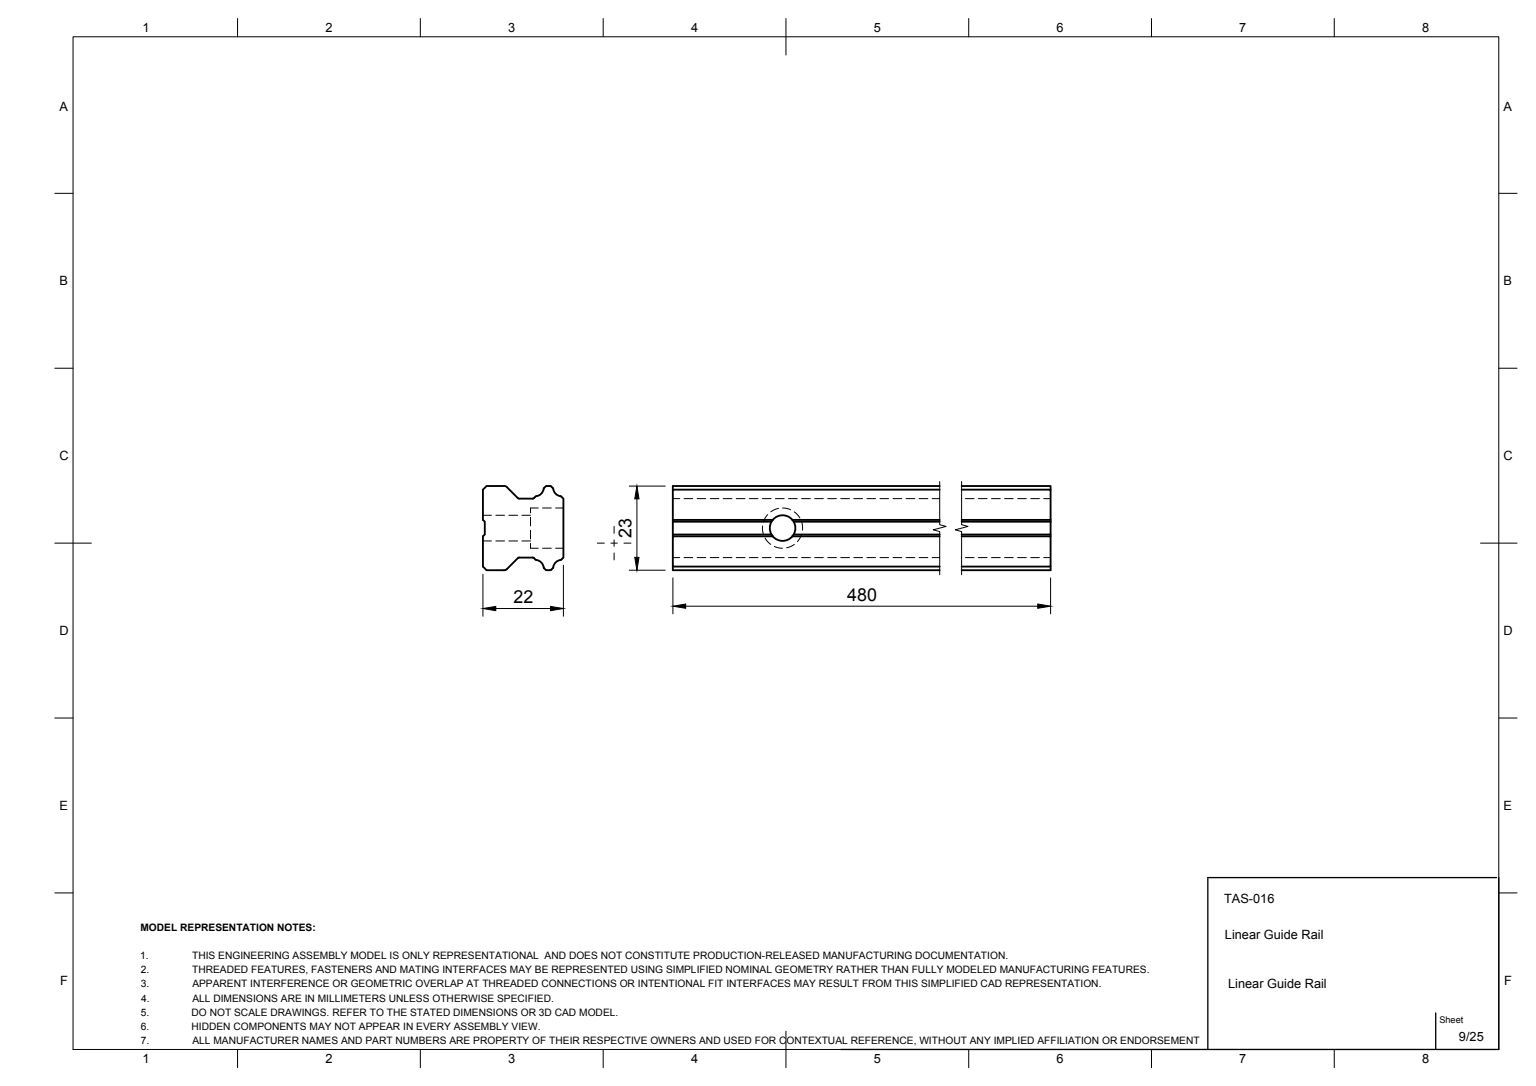
ISO-10303-21;
HEADER;
/* Generated by software containing ST-Developer
 * from STEP Tools, Inc. (www.steptools.com) 
 */

FILE_DESCRIPTION(
/* description */ ('STEP AP214'),
/* implementation_level */ '2;1');

FILE_NAME(
/* name */ 'Linear Guide Rail.step',
/* time_stamp */ '2026-11-15T14:55:55-08:00',
/* author */ (''),
/* organization */ (''),
/* preprocessor_version */ 'ST-DEVELOPER v20.2',
/* originating_system */ 'Autodesk Translation Framework v15.17.0.0',
/* authorisation */ '');

FILE_SCHEMA (('AUTOMOTIVE_DESIGN { 1 0 10303 214 3 1 1 }'));
ENDSEC;

DATA;
#10=MECHANICAL_DESIGN_GEOMETRIC_PRESENTATION_REPRESENTATION('',(#950),#57079);
#114=ELLIPSE('',#26276,4.9497474883957,3.50000001766466);
#115=ELLIPSE('',#26278,4.94974741758553,3.49999995496242);
#116=ELLIPSE('',#26282,4.94974750818554,3.50000003555096);
#117=ELLIPSE('',#26284,4.94974744933131,3.49999998268176);
#118=ELLIPSE('',#26290,4.94974743847195,3.49999997330407);
#119=ELLIPSE('',#26292,4.94974746764793,3.49999999946363);
#120=ELLIPSE('',#26296,4.94974747154346,3.5000000033075);
#121=ELLIPSE('',#26298,4.94974753359465,3.50000005774664);
#122=ELLIPSE('',#26304,4.94974746728535,3.49999999928767);
#123=ELLIPSE('',#26306,4.94974746000982,3.49999999272862);
#124=ELLIPSE('',#26310,4.94974744948699,3.49999998336686);
#125=ELLIPSE('',#26312,4.9497474011199,3.49999994011925);
#126=ELLIPSE('',#26318,4.94974750261449,3.50000003056212);
#127=ELLIPSE('',#26320,4.94974746233448,3.49999999488305);
#128=ELLIPSE('',#26324,4.94974747444535,3.50000000488897);
#129=ELLIPSE('',#26326,4.94974745285853,3.49999998629991);
#130=ELLIPSE('',#26332,4.94974749221039,3.50000002143459);
#131=ELLIPSE('',#26334,4.9497474654289,3.49999999744574);
#132=ELLIPSE('',#26338,4.94974747038,3.50000000169763);
#133=ELLIPSE('',#26340,4.94974743335947,3.49999996885897);
#134=ELLIPSE('',#26346,4.94974746422059,3.499999996325);
#135=ELLIPSE('',#26348,4.94974747922217,3.50000000966916);
#136=ELLIPSE('',#26352,4.94974747015525,3.50000000157014);
#137=ELLIPSE('',#26354,4.94974745455791,3.49999998774097);
#138=ELLIPSE('',#26360,4.94974745967519,3.49999999228821);
#139=ELLIPSE('',#26362,4.94974747586437,3.5000000067607);
#140=ELLIPSE('',#26366,4.94974746928504,3.50000000078832);
#141=ELLIPSE('',#26368,4.94974746799383,3.4999999996985);
#142=ELLIPSE('',#26374,4.94974746841778,3.50000000010074);
#143=ELLIPSE('',#26376,4.94974746853704,3.50000000020677);
#144=ELLIPSE('',#26380,4.94974746848257,3.50000000010871);
#145=ELLIPSE('',#26382,4.94974746829098,3.50000000002092);
#888=SHAPE_REPRESENTATION_RELATIONSHIP('SRR','None',#57278,#917);
#917=ADVANCED_BREP_SHAPE_REPRESENTATION('',(#987),#57070);
#950=STYLED_ITEM('',(#57444),#987);
#987=MANIFOLD_SOLID_BREP('Body1',#24550);
#1277=FACE_BOUND('',#4629,.T.);
#1278=FACE_BOUND('',#4630,.T.);
#1279=FACE_BOUND('',#4631,.T.);
#1280=FACE_BOUND('',#4632,.T.);
#1281=FACE_BOUND('',#4633,.T.);
#1282=FACE_BOUND('',#4634,.T.);
#1283=FACE_BOUND('',#4635,.T.);
#1284=FACE_BOUND('',#4636,.T.);
#1285=FACE_BOUND('',#4675,.T.);
#1286=FACE_BOUND('',#4677,.T.);
#1287=FACE_BOUND('',#4679,.T.);
#1288=FACE_BOUND('',#4681,.T.);
#1289=FACE_BOUND('',#4683,.T.);
#1290=FACE_BOUND('',#4685,.T.);
#1291=FACE_BOUND('',#4687,.T.);
#1292=FACE_BOUND('',#4689,.T.);
#1730=PLANE('',#26383);
#1731=PLANE('',#26384);
#1732=PLANE('',#26385);
#1733=PLANE('',#26386);
#1734=PLANE('',#26387);
#1735=PLANE('',#26388);
#1736=PLANE('',#26389);
#1737=PLANE('',#26390);
#1738=PLANE('',#26391);
#1739=PLANE('',#26392);
#1740=PLANE('',#26393);
#1741=PLANE('',#26394);
#1742=PLANE('',#26395);
#1743=PLANE('',#26396);
#1744=PLANE('',#26397);
#1745=PLANE('',#26398);
#1746=PLANE('',#26399);
#1747=PLANE('',#26400);
#1748=PLANE('',#26401);
#1749=PLANE('',#26402);
#1750=PLANE('',#26403);
#1751=PLANE('',#26404);
#1752=PLANE('',#26405);
#1753=PLANE('',#26406);
#1754=PLANE('',#26407);
#1755=PLANE('',#26408);
#1756=PLANE('',#26409);
#1757=PLANE('',#26432);
#1758=PLANE('',#26455);
#1759=PLANE('',#26456);
#1760=PLANE('',#26457);
#1761=PLANE('',#26458);
#1762=PLANE('',#26459);
#1763=PLANE('',#26460);
#1764=PLANE('',#26461);
#1765=PLANE('',#26462);
#1766=PLANE('',#26463);
#1767=PLANE('',#26464);
#1768=PLANE('',#26465);
#1769=PLANE('',#26466);
#1770=PLANE('',#26467);
#1771=PLANE('',#26468);
#1772=PLANE('',#26480);
#1773=PLANE('',#26481);
#1774=PLANE('',#26482);
#1775=PLANE('',#26483);
#1776=PLANE('',#26484);
#1777=PLANE('',#26496);
#1778=PLANE('',#26497);
#1779=PLANE('',#26498);
#1780=PLANE('',#26499);
#1781=PLANE('',#26500);
#1782=PLANE('',#26501);
#1783=PLANE('',#26502);
#1784=PLANE('',#26503);
#1785=PLANE('',#26504);
#1786=PLANE('',#26505);
#1787=PLANE('',#26506);
#2926=FACE_OUTER_BOUND('',#4578,.T.);
#2927=FACE_OUTER_BOUND('',#4579,.T.);
#2928=FACE_OUTER_BOUND('',#4580,.T.);
#2929=FACE_OUTER_BOUND('',#4581,.T.);
#2930=FACE_OUTER_BOUND('',#4582,.T.);
#2931=FACE_OUTER_BOUND('',#4583,.T.);
#2932=FACE_OUTER_BOUND('',#4584,.T.);
#2933=FACE_OUTER_BOUND('',#4585,.T.);
#2934=FACE_OUTER_BOUND('',#4586,.T.);
#2935=FACE_OUTER_BOUND('',#4587,.T.);
#2936=FACE_OUTER_BOUND('',#4588,.T.);
#2937=FACE_OUTER_BOUND('',#4589,.T.);
#2938=FACE_OUTER_BOUND('',#4590,.T.);
#2939=FACE_OUTER_BOUND('',#4591,.T.);
#2940=FACE_OUTER_BOUND('',#4592,.T.);
#2941=FACE_OUTER_BOUND('',#4593,.T.);
#2942=FACE_OUTER_BOUND('',#4594,.T.);
#2943=FACE_OUTER_BOUND('',#4595,.T.);
#2944=FACE_OUTER_BOUND('',#4596,.T.);
#2945=FACE_OUTER_BOUND('',#4597,.T.);
#2946=FACE_OUTER_BOUND('',#4598,.T.);
#2947=FACE_OUTER_BOUND('',#4599,.T.);
#2948=FACE_OUTER_BOUND('',#4600,.T.);
#2949=FACE_OUTER_BOUND('',#4601,.T.);
#2950=FACE_OUTER_BOUND('',#4602,.T.);
#2951=FACE_OUTER_BOUND('',#4603,.T.);
#2952=FACE_OUTER_BOUND('',#4604,.T.);
#2953=FACE_OUTER_BOUND('',#4605,.T.);
#2954=FACE_OUTER_BOUND('',#4606,.T.);
#2955=FACE_OUTER_BOUND('',#4607,.T.);
#2956=FACE_OUTER_BOUND('',#4608,.T.);
#2957=FACE_OUTER_BOUND('',#4609,.T.);
#2958=FACE_OUTER_BOUND('',#4610,.T.);
#2959=FACE_OUTER_BOUND('',#4611,.T.);
#2960=FACE_OUTER_BOUND('',#4612,.T.);
#2961=FACE_OUTER_BOUND('',#4613,.T.);
#2962=FACE_OUTER_BOUND('',#4614,.T.);
#2963=FACE_OUTER_BOUND('',#4615,.T.);
#2964=FACE_OUTER_BOUND('',#4616,.T.);
#2965=FACE_OUTER_BOUND('',#4617,.T.);
#2966=FACE_OUTER_BOUND('',#4618,.T.);
#2967=FACE_OUTER_BOUND('',#4619,.T.);
#2968=FACE_OUTER_BOUND('',#4620,.T.);
#2969=FACE_OUTER_BOUND('',#4621,.T.);
#2970=FACE_OUTER_BOUND('',#4622,.T.);
#2971=FACE_OUTER_BOUND('',#4623,.T.);
#2972=FACE_OUTER_BOUND('',#4624,.T.);
#2973=FACE_OUTER_BOUND('',#4625,.T.);
#2974=FACE_OUTER_BOUND('',#4626,.T.);
#2975=FACE_OUTER_BOUND('',#4627,.T.);
#2976=FACE_OUTER_BOUND('',#4628,.T.);
#2977=FACE_OUTER_BOUND('',#4637,.T.);
#2978=FACE_OUTER_BOUND('',#4638,.T.);
#2979=FACE_OUTER_BOUND('',#4639,.T.);
#2980=FACE_OUTER_BOUND('',#4640,.T.);
#2981=FACE_OUTER_BOUND('',#4641,.T.);
#2982=FACE_OUTER_BOUND('',#4642,.T.);
#2983=FACE_OUTER_BOUND('',#4643,.T.);
#2984=FACE_OUTER_BOUND('',#4644,.T.);
#2985=FACE_OUTER_BOUND('',#4645,.T.);
#2986=FACE_OUTER_BOUND('',#4646,.T.);
#2987=FACE_OUTER_BOUND('',#4647,.T.);
#2988=FACE_OUTER_BOUND('',#4648,.T.);
#2989=FACE_OUTER_BOUND('',#4649,.T.);
#2990=FACE_OUTER_BOUND('',#4650,.T.);
#2991=FACE_OUTER_BOUND('',#4651,.T.);
#2992=FACE_OUTER_BOUND('',#4652,.T.);
#2993=FACE_OUTER_BOUND('',#4653,.T.);
#2994=FACE_OUTER_BOUND('',#4654,.T.);
#2995=FACE_OUTER_BOUND('',#4655,.T.);
#2996=FACE_OUTER_BOUND('',#4656,.T.);
#2997=FACE_OUTER_BOUND('',#4657,.T.);
#2998=FACE_OUTER_BOUND('',#4658,.T.);
#2999=FACE_OUTER_BOUND('',#4659,.T.);
#3000=FACE_OUTER_BOUND('',#4660,.T.);
#3001=FACE_OUTER_BOUND('',#4661,.T.);
#3002=FACE_OUTER_BOUND('',#4662,.T.);
#3003=FACE_OUTER_BOUND('',#4663,.T.);
#3004=FACE_OUTER_BOUND('',#4664,.T.);
#3005=FACE_OUTER_BOUND('',#4665,.T.);
#3006=FACE_OUTER_BOUND('',#4666,.T.);
#3007=FACE_OUTER_BOUND('',#4667,.T.);
#3008=FACE_OUTER_BOUND('',#4668,.T.);
#3009=FACE_OUTER_BOUND('',#4669,.T.);
#3010=FACE_OUTER_BOUND('',#4670,.T.);
#3011=FACE_OUTER_BOUND('',#4671,.T.);
#3012=FACE_OUTER_BOUND('',#4672,.T.);
#3013=FACE_OUTER_BOUND('',#4673,.T.);
#3014=FACE_OUTER_BOUND('',#4674,.T.);
#3015=FACE_OUTER_BOUND('',#4676,.T.);
#3016=FACE_OUTER_BOUND('',#4678,.T.);
#3017=FACE_OUTER_BOUND('',#4680,.T.);
#3018=FACE_OUTER_BOUND('',#4682,.T.);
#3019=FACE_OUTER_BOUND('',#4684,.T.);
#3020=FACE_OUTER_BOUND('',#4686,.T.);
#3021=FACE_OUTER_BOUND('',#4688,.T.);
#4578=EDGE_LOOP('',(#19528,#19529,#19530,#19531));
#4579=EDGE_LOOP('',(#19532,#19533,#19534,#19535,#19536,#19537,#19538,#19539,
#19540,#19541,#19542,#19543));
#4580=EDGE_LOOP('',(#19544,#19545,#19546,#19547));
#4581=EDGE_LOOP('',(#19548,#19549,#19550,#19551,#19552,#19553,#19554,#19555,
#19556,#19557,#19558,#19559));
#4582=EDGE_LOOP('',(#19560,#19561,#19562,#19563));
#4583=EDGE_LOOP('',(#19564,#19565,#19566,#19567,#19568,#19569,#19570,#19571,
#19572,#19573,#19574,#19575));
#4584=EDGE_LOOP('',(#19576,#19577,#19578,#19579));
#4585=EDGE_LOOP('',(#19580,#19581,#19582,#19583,#19584,#19585,#19586,#19587,
#19588,#19589,#19590,#19591));
#4586=EDGE_LOOP('',(#19592,#19593,#19594,#19595));
#4587=EDGE_LOOP('',(#19596,#19597,#19598,#19599,#19600,#19601,#19602,#19603,
#19604,#19605,#19606,#19607));
#4588=EDGE_LOOP('',(#19608,#19609,#19610,#19611));
#4589=EDGE_LOOP('',(#19612,#19613,#19614,#19615,#19616,#19617,#19618,#19619,
#19620,#19621,#19622,#19623));
#4590=EDGE_LOOP('',(#19624,#19625,#19626,#19627));
#4591=EDGE_LOOP('',(#19628,#19629,#19630,#19631,#19632,#19633,#19634,#19635,
#19636,#19637,#19638,#19639));
#4592=EDGE_LOOP('',(#19640,#19641,#19642,#19643));
#4593=EDGE_LOOP('',(#19644,#19645,#19646,#19647,#19648,#19649,#19650,#19651,
#19652,#19653,#19654,#19655));
#4594=EDGE_LOOP('',(#19656,#19657,#19658,#19659));
#4595=EDGE_LOOP('',(#19660,#19661,#19662,#19663,#19664));
#4596=EDGE_LOOP('',(#19665,#19666,#19667,#19668));
#4597=EDGE_LOOP('',(#19669,#19670,#19671,#19672,#19673,#19674,#19675,#19676,
#19677,#19678,#19679,#19680,#19681,#19682,#19683,#19684,#19685,#19686,#19687,
#19688));
#4598=EDGE_LOOP('',(#19689,#19690,#19691,#19692,#19693,#19694,#19695,#19696,
#19697,#19698,#19699,#19700,#19701,#19702,#19703,#19704,#19705,#19706,#19707,
#19708));
#4599=EDGE_LOOP('',(#19709,#19710,#19711,#19712));
#4600=EDGE_LOOP('',(#19713,#19714,#19715,#19716,#19717));
#4601=EDGE_LOOP('',(#19718,#19719,#19720,#19721));
#4602=EDGE_LOOP('',(#19722,#19723,#19724,#19725));
#4603=EDGE_LOOP('',(#19726,#19727,#19728,#19729,#19730));
#4604=EDGE_LOOP('',(#19731,#19732,#19733,#19734));
#4605=EDGE_LOOP('',(#19735,#19736,#19737,#19738));
#4606=EDGE_LOOP('',(#19739,#19740,#19741,#19742));
#4607=EDGE_LOOP('',(#19743,#19744,#19745,#19746,#19747));
#4608=EDGE_LOOP('',(#19748,#19749,#19750,#19751));
#4609=EDGE_LOOP('',(#19752,#19753,#19754,#19755,#19756));
#4610=EDGE_LOOP('',(#19757,#19758,#19759,#19760));
#4611=EDGE_LOOP('',(#19761,#19762,#19763,#19764));
#4612=EDGE_LOOP('',(#19765,#19766,#19767,#19768,#19769));
#4613=EDGE_LOOP('',(#19770,#19771,#19772,#19773));
#4614=EDGE_LOOP('',(#19774,#19775,#19776,#19777));
#4615=EDGE_LOOP('',(#19778,#19779,#19780,#19781,#19782));
#4616=EDGE_LOOP('',(#19783,#19784,#19785,#19786));
#4617=EDGE_LOOP('',(#19787,#19788,#19789,#19790));
#4618=EDGE_LOOP('',(#19791,#19792,#19793,#19794));
#4619=EDGE_LOOP('',(#19795,#19796,#19797,#19798));
#4620=EDGE_LOOP('',(#19799,#19800,#19801,#19802,#19803,#19804,#19805,#19806,
#19807,#19808,#19809,#19810,#19811,#19812,#19813,#19814,#19815,#19816,#19817,
#19818,#19819,#19820,#19821,#19822,#19823,#19824,#19825,#19826,#19827,#19828,
#19829,#19830,#19831,#19832,#19833,#19834,#19835,#19836,#19837,#19838,#19839,
#19840,#19841,#19842,#19843,#19844));
#4621=EDGE_LOOP('',(#19845,#19846,#19847,#19848,#19849,#19850,#19851,#19852,
#19853,#19854,#19855,#19856,#19857,#19858,#19859,#19860,#19861,#19862,#19863,
#19864,#19865,#19866,#19867,#19868,#19869,#19870,#19871,#19872,#19873,#19874,
#19875,#19876,#19877,#19878,#19879,#19880,#19881,#19882,#19883,#19884,#19885,
#19886,#19887,#19888,#19889,#19890));
#4622=EDGE_LOOP('',(#19891,#19892,#19893,#19894));
#4623=EDGE_LOOP('',(#19895,#19896,#19897,#19898));
#4624=EDGE_LOOP('',(#19899,#19900,#19901,#19902));
#4625=EDGE_LOOP('',(#19903,#19904,#19905,#19906));
#4626=EDGE_LOOP('',(#19907,#19908,#19909,#19910));
#4627=EDGE_LOOP('',(#19911,#19912,#19913,#19914));
#4628=EDGE_LOOP('',(#19915,#19916,#19917,#19918));
#4629=EDGE_LOOP('',(#19919));
#4630=EDGE_LOOP('',(#19920));
#4631=EDGE_LOOP('',(#19921));
#4632=EDGE_LOOP('',(#19922));
#4633=EDGE_LOOP('',(#19923));
#4634=EDGE_LOOP('',(#19924));
#4635=EDGE_LOOP('',(#19925));
#4636=EDGE_LOOP('',(#19926));
#4637=EDGE_LOOP('',(#19927,#19928,#19929,#19930));
#4638=EDGE_LOOP('',(#19931,#19932,#19933,#19934));
#4639=EDGE_LOOP('',(#19935,#19936,#19937,#19938));
#4640=EDGE_LOOP('',(#19939,#19940,#19941,#19942));
#4641=EDGE_LOOP('',(#19943,#19944,#19945,#19946));
#4642=EDGE_LOOP('',(#19947,#19948,#19949,#19950));
#4643=EDGE_LOOP('',(#19951,#19952,#19953,#19954));
#4644=EDGE_LOOP('',(#19955,#19956,#19957,#19958));
#4645=EDGE_LOOP('',(#19959,#19960,#19961,#19962));
#4646=EDGE_LOOP('',(#19963,#19964,#19965,#19966));
#4647=EDGE_LOOP('',(#19967,#19968,#19969,#19970));
#4648=EDGE_LOOP('',(#19971,#19972,#19973,#19974));
#4649=EDGE_LOOP('',(#19975,#19976,#19977,#19978));
#4650=EDGE_LOOP('',(#19979,#19980,#19981,#19982));
#4651=EDGE_LOOP('',(#19983,#19984,#19985,#19986));
#4652=EDGE_LOOP('',(#19987,#19988,#19989,#19990));
#4653=EDGE_LOOP('',(#19991,#19992,#19993,#19994));
#4654=EDGE_LOOP('',(#19995,#19996,#19997,#19998));
#4655=EDGE_LOOP('',(#19999,#20000,#20001,#20002));
#4656=EDGE_LOOP('',(#20003,#20004,#20005,#20006));
#4657=EDGE_LOOP('',(#20007,#20008,#20009,#20010));
#4658=EDGE_LOOP('',(#20011,#20012,#20013,#20014));
#4659=EDGE_LOOP('',(#20015,#20016,#20017,#20018));
#4660=EDGE_LOOP('',(#20019,#20020,#20021,#20022));
#4661=EDGE_LOOP('',(#20023,#20024,#20025,#20026));
#4662=EDGE_LOOP('',(#20027,#20028,#20029,#20030));
#4663=EDGE_LOOP('',(#20031,#20032,#20033,#20034));
#4664=EDGE_LOOP('',(#20035,#20036,#20037,#20038));
#4665=EDGE_LOOP('',(#20039,#20040,#20041,#20042));
#4666=EDGE_LOOP('',(#20043,#20044,#20045,#20046));
#4667=EDGE_LOOP('',(#20047,#20048,#20049,#20050));
#4668=EDGE_LOOP('',(#20051,#20052,#20053,#20054));
#4669=EDGE_LOOP('',(#20055,#20056,#20057,#20058));
#4670=EDGE_LOOP('',(#20059,#20060,#20061,#20062));
#4671=EDGE_LOOP('',(#20063,#20064,#20065,#20066));
#4672=EDGE_LOOP('',(#20067,#20068,#20069,#20070,#20071));
#4673=EDGE_LOOP('',(#20072,#20073,#20074,#20075));
#4674=EDGE_LOOP('',(#20076));
#4675=EDGE_LOOP('',(#20077));
#4676=EDGE_LOOP('',(#20078));
#4677=EDGE_LOOP('',(#20079));
#4678=EDGE_LOOP('',(#20080));
#4679=EDGE_LOOP('',(#20081));
#4680=EDGE_LOOP('',(#20082));
#4681=EDGE_LOOP('',(#20083));
#4682=EDGE_LOOP('',(#20084));
#4683=EDGE_LOOP('',(#20085));
#4684=EDGE_LOOP('',(#20086));
#4685=EDGE_LOOP('',(#20087));
#4686=EDGE_LOOP('',(#20088));
#4687=EDGE_LOOP('',(#20089));
#4688=EDGE_LOOP('',(#20090));
#4689=EDGE_LOOP('',(#20091));
#6163=LINE('',#53474,#8130);
#6164=LINE('',#53489,#8131);
#6165=LINE('',#53502,#8132);
#6166=LINE('',#53517,#8133);
#6167=LINE('',#53530,#8134);
#6168=LINE('',#53545,#8135);
#6169=LINE('',#53558,#8136);
#6170=LINE('',#53573,#8137);
#6171=LINE('',#53586,#8138);
#6172=LINE('',#53601,#8139);
#6173=LINE('',#53614,#8140);
#6174=LINE('',#53629,#8141);
#6175=LINE('',#53642,#8142);
#6176=LINE('',#53657,#8143);
#6177=LINE('',#53670,#8144);
#6178=LINE('',#53685,#8145);
#6179=LINE('',#53696,#8146);
#6180=LINE('',#53698,#8147);
#6181=LINE('',#53699,#8148);
#6182=LINE('',#53701,#8149);
#6183=LINE('',#53702,#8150);
#6184=LINE('',#53704,#8151);
#6185=LINE('',#53706,#8152);
#6186=LINE('',#53707,#8153);
#6187=LINE('',#53708,#8154);
#6188=LINE('',#53709,#8155);
#6189=LINE('',#53710,#8156);
#6190=LINE('',#53711,#8157);
#6191=LINE('',#53712,#8158);
#6192=LINE('',#53714,#8159);
#6193=LINE('',#53716,#8160);
#6194=LINE('',#53718,#8161);
#6195=LINE('',#53719,#8162);
#6196=LINE('',#53722,#8163);
#6197=LINE('',#53724,#8164);
#6198=LINE('',#53726,#8165);
#6199=LINE('',#53728,#8166);
#6200=LINE('',#53729,#8167);
#6201=LINE('',#53730,#8168);
#6202=LINE('',#53731,#8169);
#6203=LINE('',#53732,#8170);
#6204=LINE('',#53733,#8171);
#6205=LINE('',#53734,#8172);
#6206=LINE('',#53735,#8173);
#6207=LINE('',#53738,#8174);
#6208=LINE('',#53739,#8175);
#6209=LINE('',#53743,#8176);
#6210=LINE('',#53744,#8177);
#6211=LINE('',#53748,#8178);
#6212=LINE('',#53750,#8179);
#6213=LINE('',#53753,#8180);
#6214=LINE('',#53754,#8181);
#6215=LINE('',#53758,#8182);
#6216=LINE('',#53759,#8183);
#6217=LINE('',#53763,#8184);
#6218=LINE('',#53764,#8185);
#6219=LINE('',#53769,#8186);
#6220=LINE('',#53771,#8187);
#6221=LINE('',#53772,#8188);
#6222=LINE('',#53774,#8189);
#6223=LINE('',#53777,#8190);
#6224=LINE('',#53779,#8191);
#6225=LINE('',#53783,#8192);
#6226=LINE('',#53787,#8193);
#6227=LINE('',#53791,#8194);
#6228=LINE('',#53799,#8195);
#6229=LINE('',#53803,#8196);
#6230=LINE('',#53807,#8197);
#6231=LINE('',#53815,#8198);
#6232=LINE('',#53817,#8199);
#6233=LINE('',#53819,#8200);
#6234=LINE('',#53827,#8201);
#6235=LINE('',#53831,#8202);
#6236=LINE('',#53835,#8203);
#6237=LINE('',#53843,#8204);
#6238=LINE('',#53847,#8205);
#6239=LINE('',#53851,#8206);
#6240=LINE('',#53855,#8207);
#6241=LINE('',#53856,#8208);
#6242=LINE('',#53858,#8209);
#6243=LINE('',#53859,#8210);
#6244=LINE('',#53861,#8211);
#6245=LINE('',#53863,#8212);
#6246=LINE('',#53865,#8213);
#6247=LINE('',#53869,#8214);
#6248=LINE('',#53873,#8215);
#6249=LINE('',#53877,#8216);
#6250=LINE('',#53885,#8217);
#6251=LINE('',#53889,#8218);
#6252=LINE('',#53893,#8219);
#6253=LINE('',#53901,#8220);
#6254=LINE('',#53903,#8221);
#6255=LINE('',#53905,#8222);
#6256=LINE('',#53913,#8223);
#6257=LINE('',#53917,#8224);
#6258=LINE('',#53921,#8225);
#6259=LINE('',#53929,#8226);
#6260=LINE('',#53933,#8227);
#6261=LINE('',#53937,#8228);
#6262=LINE('',#53941,#8229);
#6263=LINE('',#53942,#8230);
#6264=LINE('',#53944,#8231);
#6265=LINE('',#53945,#8232);
#6266=LINE('',#53947,#8233);
#6267=LINE('',#53948,#8234);
#6268=LINE('',#53950,#8235);
#6269=LINE('',#53951,#8236);
#6270=LINE('',#53953,#8237);
#6271=LINE('',#53954,#8238);
#6272=LINE('',#53956,#8239);
#6273=LINE('',#53957,#8240);
#6274=LINE('',#53959,#8241);
#6275=LINE('',#53960,#8242);
#6276=LINE('',#53962,#8243);
#6277=LINE('',#53964,#8244);
#6278=LINE('',#53966,#8245);
#6279=LINE('',#53968,#8246);
#6280=LINE('',#53969,#8247);
#6281=LINE('',#53971,#8248);
#6282=LINE('',#53972,#8249);
#6283=LINE('',#53974,#8250);
#6284=LINE('',#53975,#8251);
#6285=LINE('',#53977,#8252);
#6286=LINE('',#53978,#8253);
#6287=LINE('',#53980,#8254);
#6288=LINE('',#53982,#8255);
#6289=LINE('',#53983,#8256);
#6290=LINE('',#53985,#8257);
#6291=LINE('',#53986,#8258);
#6292=LINE('',#53997,#8259);
#6293=LINE('',#53998,#8260);
#6294=LINE('',#54000,#8261);
#6295=LINE('',#54001,#8262);
#6296=LINE('',#54003,#8263);
#6297=LINE('',#54004,#8264);
#6298=LINE('',#54006,#8265);
#6299=LINE('',#54007,#8266);
#6300=LINE('',#54010,#8267);
#6301=LINE('',#54011,#8268);
#6302=LINE('',#54013,#8269);
#6303=LINE('',#54014,#8270);
#6304=LINE('',#54026,#8271);
#8130=VECTOR('',#31169,5.50000000000001);
#8131=VECTOR('',#31184,3.5);
#8132=VECTOR('',#31199,5.50000000000001);
#8133=VECTOR('',#31214,3.5);
#8134=VECTOR('',#31229,5.50000000000001);
#8135=VECTOR('',#31244,3.5);
#8136=VECTOR('',#31259,5.50000000000001);
#8137=VECTOR('',#31274,3.5);
#8138=VECTOR('',#31289,5.50000000000001);
#8139=VECTOR('',#31304,3.5);
#8140=VECTOR('',#31319,5.50000000000001);
#8141=VECTOR('',#31334,3.5);
#8142=VECTOR('',#31349,5.5);
#8143=VECTOR('',#31364,3.5);
#8144=VECTOR('',#31379,5.5);
#8145=VECTOR('',#31394,3.5);
#8146=VECTOR('',#31407,1000.);
#8147=VECTOR('',#31408,1000.);
#8148=VECTOR('',#31409,1000.);
#8149=VECTOR('',#31412,1000.);
#8150=VECTOR('',#31413,1000.);
#8151=VECTOR('',#31416,1000.);
#8152=VECTOR('',#31419,1000.);
#8153=VECTOR('',#31420,1000.);
#8154=VECTOR('',#31421,1000.);
#8155=VECTOR('',#31422,1000.);
#8156=VECTOR('',#31423,1000.);
#8157=VECTOR('',#31424,1000.);
#8158=VECTOR('',#31425,1000.);
#8159=VECTOR('',#31426,1000.);
#8160=VECTOR('',#31427,1000.);
#8161=VECTOR('',#31428,1000.);
#8162=VECTOR('',#31429,1000.);
#8163=VECTOR('',#31432,1000.);
#8164=VECTOR('',#31433,1000.);
#8165=VECTOR('',#31434,1000.);
#8166=VECTOR('',#31435,1000.);
#8167=VECTOR('',#31436,1000.);
#8168=VECTOR('',#31437,1000.);
#8169=VECTOR('',#31438,1000.);
#8170=VECTOR('',#31439,1000.);
#8171=VECTOR('',#31440,1000.);
#8172=VECTOR('',#31441,1000.);
#8173=VECTOR('',#31442,1000.);
#8174=VECTOR('',#31447,1000.);
#8175=VECTOR('',#31448,1000.);
#8176=VECTOR('',#31455,1000.);
#8177=VECTOR('',#31456,1000.);
#8178=VECTOR('',#31463,1000.);
#8179=VECTOR('',#31466,1000.);
#8180=VECTOR('',#31471,1000.);
#8181=VECTOR('',#31472,1000.);
#8182=VECTOR('',#31479,1000.);
#8183=VECTOR('',#31480,1000.);
#8184=VECTOR('',#31487,1000.);
#8185=VECTOR('',#31488,1000.);
#8186=VECTOR('',#31495,1000.);
#8187=VECTOR('',#31496,1000.);
#8188=VECTOR('',#31497,1000.);
#8189=VECTOR('',#31500,1000.);
#8190=VECTOR('',#31503,1000.);
#8191=VECTOR('',#31504,1000.);
#8192=VECTOR('',#31507,1000.);
#8193=VECTOR('',#31510,1000.);
#8194=VECTOR('',#31513,1000.);
#8195=VECTOR('',#31520,1000.);
#8196=VECTOR('',#31523,1000.);
#8197=VECTOR('',#31526,1000.);
#8198=VECTOR('',#31533,1000.);
#8199=VECTOR('',#31534,1000.);
#8200=VECTOR('',#31535,1000.);
#8201=VECTOR('',#31542,1000.);
#8202=VECTOR('',#31545,1000.);
#8203=VECTOR('',#31548,1000.);
#8204=VECTOR('',#31555,1000.);
#8205=VECTOR('',#31558,1000.);
#8206=VECTOR('',#31561,1000.);
#8207=VECTOR('',#31564,1000.);
#8208=VECTOR('',#31565,1000.);
#8209=VECTOR('',#31566,1000.);
#8210=VECTOR('',#31567,1000.);
#8211=VECTOR('',#31570,1000.);
#8212=VECTOR('',#31571,1000.);
#8213=VECTOR('',#31572,1000.);
#8214=VECTOR('',#31575,1000.);
#8215=VECTOR('',#31578,1000.);
#8216=VECTOR('',#31581,1000.);
#8217=VECTOR('',#31588,1000.);
#8218=VECTOR('',#31591,1000.);
#8219=VECTOR('',#31594,1000.);
#8220=VECTOR('',#31601,1000.);
#8221=VECTOR('',#31602,1000.);
#8222=VECTOR('',#31603,1000.);
#8223=VECTOR('',#31610,1000.);
#8224=VECTOR('',#31613,1000.);
#8225=VECTOR('',#31616,1000.);
#8226=VECTOR('',#31623,1000.);
#8227=VECTOR('',#31626,1000.);
#8228=VECTOR('',#31629,1000.);
#8229=VECTOR('',#31632,1000.);
#8230=VECTOR('',#31633,1000.);
#8231=VECTOR('',#31636,1000.);
#8232=VECTOR('',#31637,1000.);
#8233=VECTOR('',#31640,1000.);
#8234=VECTOR('',#31641,1000.);
#8235=VECTOR('',#31644,1000.);
#8236=VECTOR('',#31645,1000.);
#8237=VECTOR('',#31648,1000.);
#8238=VECTOR('',#31649,1000.);
#8239=VECTOR('',#31652,1000.);
#8240=VECTOR('',#31653,1000.);
#8241=VECTOR('',#31656,1000.);
#8242=VECTOR('',#31657,1000.);
#8243=VECTOR('',#31660,1000.);
#8244=VECTOR('',#31663,1000.);
#8245=VECTOR('',#31666,1000.);
#8246=VECTOR('',#31669,1000.);
#8247=VECTOR('',#31670,1000.);
#8248=VECTOR('',#31673,1000.);
#8249=VECTOR('',#31674,1000.);
#8250=VECTOR('',#31677,1000.);
#8251=VECTOR('',#31678,1000.);
#8252=VECTOR('',#31681,1000.);
#8253=VECTOR('',#31682,1000.);
#8254=VECTOR('',#31685,1000.);
#8255=VECTOR('',#31688,1000.);
#8256=VECTOR('',#31689,1000.);
#8257=VECTOR('',#31692,1000.);
#8258=VECTOR('',#31693,1000.);
#8259=VECTOR('',#31714,1000.);
#8260=VECTOR('',#31715,1000.);
#8261=VECTOR('',#31718,1000.);
#8262=VECTOR('',#31719,1000.);
#8263=VECTOR('',#31722,1000.);
#8264=VECTOR('',#31723,1000.);
#8265=VECTOR('',#31726,1000.);
#8266=VECTOR('',#31727,1000.);
#8267=VECTOR('',#31732,1000.);
#8268=VECTOR('',#31733,1000.);
#8269=VECTOR('',#31736,1000.);
#8270=VECTOR('',#31737,1000.);
#8271=VECTOR('',#31760,1000.);
#9808=CIRCLE('',#26272,5.50000000000001);
#9809=CIRCLE('',#26273,5.50000000000001);
#9810=CIRCLE('',#26275,3.5);
#9811=CIRCLE('',#26277,3.5);
#9812=CIRCLE('',#26279,3.5);
#9813=CIRCLE('',#26280,3.5);
#9814=CIRCLE('',#26281,3.5);
#9815=CIRCLE('',#26283,3.5);
#9816=CIRCLE('',#26286,5.50000000000001);
#9817=CIRCLE('',#26287,5.50000000000001);
#9818=CIRCLE('',#26289,3.5);
#9819=CIRCLE('',#26291,3.5);
#9820=CIRCLE('',#26293,3.5);
#9821=CIRCLE('',#26294,3.5);
#9822=CIRCLE('',#26295,3.5);
#9823=CIRCLE('',#26297,3.5);
#9824=CIRCLE('',#26300,5.50000000000001);
#9825=CIRCLE('',#26301,5.50000000000001);
#9826=CIRCLE('',#26303,3.5);
#9827=CIRCLE('',#26305,3.5);
#9828=CIRCLE('',#26307,3.5);
#9829=CIRCLE('',#26308,3.5);
#9830=CIRCLE('',#26309,3.5);
#9831=CIRCLE('',#26311,3.5);
#9832=CIRCLE('',#26314,5.50000000000001);
#9833=CIRCLE('',#26315,5.50000000000001);
#9834=CIRCLE('',#26317,3.5);
#9835=CIRCLE('',#26319,3.5);
#9836=CIRCLE('',#26321,3.5);
#9837=CIRCLE('',#26322,3.5);
#9838=CIRCLE('',#26323,3.5);
#9839=CIRCLE('',#26325,3.5);
#9840=CIRCLE('',#26328,5.50000000000001);
#9841=CIRCLE('',#26329,5.50000000000001);
#9842=CIRCLE('',#26331,3.5);
#9843=CIRCLE('',#26333,3.5);
#9844=CIRCLE('',#26335,3.5);
#9845=CIRCLE('',#26336,3.5);
#9846=CIRCLE('',#26337,3.5);
#9847=CIRCLE('',#26339,3.5);
#9848=CIRCLE('',#26342,5.50000000000001);
#9849=CIRCLE('',#26343,5.50000000000001);
#9850=CIRCLE('',#26345,3.5);
#9851=CIRCLE('',#26347,3.49999999999999);
#9852=CIRCLE('',#26349,3.5);
#9853=CIRCLE('',#26350,3.5);
#9854=CIRCLE('',#26351,3.5);
#9855=CIRCLE('',#26353,3.49999999999999);
#9856=CIRCLE('',#26356,5.5);
#9857=CIRCLE('',#26357,5.5);
#9858=CIRCLE('',#26359,3.5);
#9859=CIRCLE('',#26361,3.5);
#9860=CIRCLE('',#26363,3.5);
#9861=CIRCLE('',#26364,3.5);
#9862=CIRCLE('',#26365,3.5);
#9863=CIRCLE('',#26367,3.5);
#9864=CIRCLE('',#26370,5.5);
#9865=CIRCLE('',#26371,5.5);
#9866=CIRCLE('',#26373,3.5);
#9867=CIRCLE('',#26375,3.49999999999999);
#9868=CIRCLE('',#26377,3.5);
#9869=CIRCLE('',#26378,3.5);
#9870=CIRCLE('',#26379,3.5);
#9871=CIRCLE('',#26381,3.49999999999999);
#9872=CIRCLE('',#26410,0.999999999999999);
#9873=CIRCLE('',#26411,0.5);
#9874=CIRCLE('',#26412,0.5);
#9875=CIRCLE('',#26413,0.5);
#9876=CIRCLE('',#26414,2.3);
#9877=CIRCLE('',#26415,0.5);
#9878=CIRCLE('',#26416,0.5);
#9879=CIRCLE('',#26417,0.5);
#9880=CIRCLE('',#26418,0.5);
#9881=CIRCLE('',#26419,2.3);
#9882=CIRCLE('',#26420,0.5);
#9883=CIRCLE('',#26421,0.5);
#9884=CIRCLE('',#26422,2.3);
#9885=CIRCLE('',#26423,0.5);
#9886=CIRCLE('',#26424,0.5);
#9887=CIRCLE('',#26425,0.5);
#9888=CIRCLE('',#26426,0.5);
#9889=CIRCLE('',#26427,2.3);
#9890=CIRCLE('',#26428,0.5);
#9891=CIRCLE('',#26429,0.5);
#9892=CIRCLE('',#26430,0.5);
#9893=CIRCLE('',#26431,0.999999999999999);
#9894=CIRCLE('',#26433,0.999999999999999);
#9895=CIRCLE('',#26434,0.5);
#9896=CIRCLE('',#26435,0.5);
#9897=CIRCLE('',#26436,0.5);
#9898=CIRCLE('',#26437,2.3);
#9899=CIRCLE('',#26438,0.5);
#9900=CIRCLE('',#26439,0.5);
#9901=CIRCLE('',#26440,0.5);
#9902=CIRCLE('',#26441,0.5);
#9903=CIRCLE('',#26442,2.3);
#9904=CIRCLE('',#26443,0.5);
#9905=CIRCLE('',#26444,0.5);
#9906=CIRCLE('',#26445,2.3);
#9907=CIRCLE('',#26446,0.5);
#9908=CIRCLE('',#26447,0.5);
#9909=CIRCLE('',#26448,0.5);
#9910=CIRCLE('',#26449,0.5);
#9911=CIRCLE('',#26450,2.3);
#9912=CIRCLE('',#26451,0.5);
#9913=CIRCLE('',#26452,0.5);
#9914=CIRCLE('',#26453,0.5);
#9915=CIRCLE('',#26454,0.999999999999999);
#11441=VERTEX_POINT('',#53471);
#11442=VERTEX_POINT('',#53473);
#11443=VERTEX_POINT('',#53477);
#11444=VERTEX_POINT('',#53478);
#11445=VERTEX_POINT('',#53480);
#11446=VERTEX_POINT('',#53482);
#11447=VERTEX_POINT('',#53484);
#11448=VERTEX_POINT('',#53486);
#11449=VERTEX_POINT('',#53488);
#11450=VERTEX_POINT('',#53491);
#11451=VERTEX_POINT('',#53493);
#11452=VERTEX_POINT('',#53495);
#11453=VERTEX_POINT('',#53499);
#11454=VERTEX_POINT('',#53501);
#11455=VERTEX_POINT('',#53505);
#11456=VERTEX_POINT('',#53506);
#11457=VERTEX_POINT('',#53508);
#11458=VERTEX_POINT('',#53510);
#11459=VERTEX_POINT('',#53512);
#11460=VERTEX_POINT('',#53514);
#11461=VERTEX_POINT('',#53516);
#11462=VERTEX_POINT('',#53519);
#11463=VERTEX_POINT('',#53521);
#11464=VERTEX_POINT('',#53523);
#11465=VERTEX_POINT('',#53527);
#11466=VERTEX_POINT('',#53529);
#11467=VERTEX_POINT('',#53533);
#11468=VERTEX_POINT('',#53534);
#11469=VERTEX_POINT('',#53536);
#11470=VERTEX_POINT('',#53538);
#11471=VERTEX_POINT('',#53540);
#11472=VERTEX_POINT('',#53542);
#11473=VERTEX_POINT('',#53544);
#11474=VERTEX_POINT('',#53547);
#11475=VERTEX_POINT('',#53549);
#11476=VERTEX_POINT('',#53551);
#11477=VERTEX_POINT('',#53555);
#11478=VERTEX_POINT('',#53557);
#11479=VERTEX_POINT('',#53561);
#11480=VERTEX_POINT('',#53562);
#11481=VERTEX_POINT('',#53564);
#11482=VERTEX_POINT('',#53566);
#11483=VERTEX_POINT('',#53568);
#11484=VERTEX_POINT('',#53570);
#11485=VERTEX_POINT('',#53572);
#11486=VERTEX_POINT('',#53575);
#11487=VERTEX_POINT('',#53577);
#11488=VERTEX_POINT('',#53579);
#11489=VERTEX_POINT('',#53583);
#11490=VERTEX_POINT('',#53585);
#11491=VERTEX_POINT('',#53589);
#11492=VERTEX_POINT('',#53590);
#11493=VERTEX_POINT('',#53592);
#11494=VERTEX_POINT('',#53594);
#11495=VERTEX_POINT('',#53596);
#11496=VERTEX_POINT('',#53598);
#11497=VERTEX_POINT('',#53600);
#11498=VERTEX_POINT('',#53603);
#11499=VERTEX_POINT('',#53605);
#11500=VERTEX_POINT('',#53607);
#11501=VERTEX_POINT('',#53611);
#11502=VERTEX_POINT('',#53613);
#11503=VERTEX_POINT('',#53617);
#11504=VERTEX_POINT('',#53618);
#11505=VERTEX_POINT('',#53620);
#11506=VERTEX_POINT('',#53622);
#11507=VERTEX_POINT('',#53624);
#11508=VERTEX_POINT('',#53626);
#11509=VERTEX_POINT('',#53628);
#11510=VERTEX_POINT('',#53631);
#11511=VERTEX_POINT('',#53633);
#11512=VERTEX_POINT('',#53635);
#11513=VERTEX_POINT('',#53639);
#11514=VERTEX_POINT('',#53641);
#11515=VERTEX_POINT('',#53645);
#11516=VERTEX_POINT('',#53646);
#11517=VERTEX_POINT('',#53648);
#11518=VERTEX_POINT('',#53650);
#11519=VERTEX_POINT('',#53652);
#11520=VERTEX_POINT('',#53654);
#11521=VERTEX_POINT('',#53656);
#11522=VERTEX_POINT('',#53659);
#11523=VERTEX_POINT('',#53661);
#11524=VERTEX_POINT('',#53663);
#11525=VERTEX_POINT('',#53667);
#11526=VERTEX_POINT('',#53669);
#11527=VERTEX_POINT('',#53673);
#11528=VERTEX_POINT('',#53674);
#11529=VERTEX_POINT('',#53676);
#11530=VERTEX_POINT('',#53678);
#11531=VERTEX_POINT('',#53680);
#11532=VERTEX_POINT('',#53682);
#11533=VERTEX_POINT('',#53684);
#11534=VERTEX_POINT('',#53687);
#11535=VERTEX_POINT('',#53689);
#11536=VERTEX_POINT('',#53691);
#11537=VERTEX_POINT('',#53695);
#11538=VERTEX_POINT('',#53697);
#11539=VERTEX_POINT('',#53713);
#11540=VERTEX_POINT('',#53715);
#11541=VERTEX_POINT('',#53717);
#11542=VERTEX_POINT('',#53721);
#11543=VERTEX_POINT('',#53723);
#11544=VERTEX_POINT('',#53725);
#11545=VERTEX_POINT('',#53727);
#11546=VERTEX_POINT('',#53768);
#11547=VERTEX_POINT('',#53770);
#11548=VERTEX_POINT('',#53776);
#11549=VERTEX_POINT('',#53778);
#11550=VERTEX_POINT('',#53780);
#11551=VERTEX_POINT('',#53782);
#11552=VERTEX_POINT('',#53784);
#11553=VERTEX_POINT('',#53786);
#11554=VERTEX_POINT('',#53788);
#11555=VERTEX_POINT('',#53790);
#11556=VERTEX_POINT('',#53792);
#11557=VERTEX_POINT('',#53794);
#11558=VERTEX_POINT('',#53796);
#11559=VERTEX_POINT('',#53798);
#11560=VERTEX_POINT('',#53800);
#11561=VERTEX_POINT('',#53802);
#11562=VERTEX_POINT('',#53804);
#11563=VERTEX_POINT('',#53806);
#11564=VERTEX_POINT('',#53808);
#11565=VERTEX_POINT('',#53810);
#11566=VERTEX_POINT('',#53812);
#11567=VERTEX_POINT('',#53814);
#11568=VERTEX_POINT('',#53816);
#11569=VERTEX_POINT('',#53818);
#11570=VERTEX_POINT('',#53820);
#11571=VERTEX_POINT('',#53822);
#11572=VERTEX_POINT('',#53824);
#11573=VERTEX_POINT('',#53826);
#11574=VERTEX_POINT('',#53828);
#11575=VERTEX_POINT('',#53830);
#11576=VERTEX_POINT('',#53832);
#11577=VERTEX_POINT('',#53834);
#11578=VERTEX_POINT('',#53836);
#11579=VERTEX_POINT('',#53838);
#11580=VERTEX_POINT('',#53840);
#11581=VERTEX_POINT('',#53842);
#11582=VERTEX_POINT('',#53844);
#11583=VERTEX_POINT('',#53846);
#11584=VERTEX_POINT('',#53848);
#11585=VERTEX_POINT('',#53850);
#11586=VERTEX_POINT('',#53852);
#11587=VERTEX_POINT('',#53854);
#11588=VERTEX_POINT('',#53857);
#11589=VERTEX_POINT('',#53862);
#11590=VERTEX_POINT('',#53864);
#11591=VERTEX_POINT('',#53866);
#11592=VERTEX_POINT('',#53868);
#11593=VERTEX_POINT('',#53870);
#11594=VERTEX_POINT('',#53872);
#11595=VERTEX_POINT('',#53874);
#11596=VERTEX_POINT('',#53876);
#11597=VERTEX_POINT('',#53878);
#11598=VERTEX_POINT('',#53880);
#11599=VERTEX_POINT('',#53882);
#11600=VERTEX_POINT('',#53884);
#11601=VERTEX_POINT('',#53886);
#11602=VERTEX_POINT('',#53888);
#11603=VERTEX_POINT('',#53890);
#11604=VERTEX_POINT('',#53892);
#11605=VERTEX_POINT('',#53894);
#11606=VERTEX_POINT('',#53896);
#11607=VERTEX_POINT('',#53898);
#11608=VERTEX_POINT('',#53900);
#11609=VERTEX_POINT('',#53902);
#11610=VERTEX_POINT('',#53904);
#11611=VERTEX_POINT('',#53906);
#11612=VERTEX_POINT('',#53908);
#11613=VERTEX_POINT('',#53910);
#11614=VERTEX_POINT('',#53912);
#11615=VERTEX_POINT('',#53914);
#11616=VERTEX_POINT('',#53916);
#11617=VERTEX_POINT('',#53918);
#11618=VERTEX_POINT('',#53920);
#11619=VERTEX_POINT('',#53922);
#11620=VERTEX_POINT('',#53924);
#11621=VERTEX_POINT('',#53926);
#11622=VERTEX_POINT('',#53928);
#11623=VERTEX_POINT('',#53930);
#11624=VERTEX_POINT('',#53932);
#11625=VERTEX_POINT('',#53934);
#11626=VERTEX_POINT('',#53936);
#11627=VERTEX_POINT('',#53938);
#11628=VERTEX_POINT('',#53940);
#14309=EDGE_CURVE('',#11441,#11441,#9808,.T.);
#14310=EDGE_CURVE('',#11441,#11442,#6163,.T.);
#14311=EDGE_CURVE('',#11442,#11442,#9809,.T.);
#14312=EDGE_CURVE('',#11443,#11444,#9810,.T.);
#14313=EDGE_CURVE('',#11445,#11443,#114,.T.);
#14314=EDGE_CURVE('',#11446,#11445,#9811,.T.);
#14315=EDGE_CURVE('',#11447,#11446,#115,.T.);
#14316=EDGE_CURVE('',#11448,#11447,#9812,.T.);
#14317=EDGE_CURVE('',#11448,#11449,#6164,.T.);
#14318=EDGE_CURVE('',#11449,#11449,#9813,.T.);
#14319=EDGE_CURVE('',#11450,#11448,#9814,.T.);
#14320=EDGE_CURVE('',#11451,#11450,#116,.T.);
#14321=EDGE_CURVE('',#11452,#11451,#9815,.T.);
#14322=EDGE_CURVE('',#11444,#11452,#117,.T.);
#14323=EDGE_CURVE('',#11453,#11453,#9816,.T.);
#14324=EDGE_CURVE('',#11453,#11454,#6165,.T.);
#14325=EDGE_CURVE('',#11454,#11454,#9817,.T.);
#14326=EDGE_CURVE('',#11455,#11456,#9818,.T.);
#14327=EDGE_CURVE('',#11457,#11455,#118,.T.);
#14328=EDGE_CURVE('',#11458,#11457,#9819,.T.);
#14329=EDGE_CURVE('',#11459,#11458,#119,.T.);
#14330=EDGE_CURVE('',#11460,#11459,#9820,.T.);
#14331=EDGE_CURVE('',#11460,#11461,#6166,.T.);
#14332=EDGE_CURVE('',#11461,#11461,#9821,.T.);
#14333=EDGE_CURVE('',#11462,#11460,#9822,.T.);
#14334=EDGE_CURVE('',#11463,#11462,#120,.T.);
#14335=EDGE_CURVE('',#11464,#11463,#9823,.T.);
#14336=EDGE_CURVE('',#11456,#11464,#121,.T.);
#14337=EDGE_CURVE('',#11465,#11465,#9824,.T.);
#14338=EDGE_CURVE('',#11465,#11466,#6167,.T.);
#14339=EDGE_CURVE('',#11466,#11466,#9825,.T.);
#14340=EDGE_CURVE('',#11467,#11468,#9826,.T.);
#14341=EDGE_CURVE('',#11469,#11467,#122,.T.);
#14342=EDGE_CURVE('',#11470,#11469,#9827,.T.);
#14343=EDGE_CURVE('',#11471,#11470,#123,.T.);
#14344=EDGE_CURVE('',#11472,#11471,#9828,.T.);
#14345=EDGE_CURVE('',#11472,#11473,#6168,.T.);
#14346=EDGE_CURVE('',#11473,#11473,#9829,.T.);
#14347=EDGE_CURVE('',#11474,#11472,#9830,.T.);
#14348=EDGE_CURVE('',#11475,#11474,#124,.T.);
#14349=EDGE_CURVE('',#11476,#11475,#9831,.T.);
#14350=EDGE_CURVE('',#11468,#11476,#125,.T.);
#14351=EDGE_CURVE('',#11477,#11477,#9832,.T.);
#14352=EDGE_CURVE('',#11477,#11478,#6169,.T.);
#14353=EDGE_CURVE('',#11478,#11478,#9833,.T.);
#14354=EDGE_CURVE('',#11479,#11480,#9834,.T.);
#14355=EDGE_CURVE('',#11481,#11479,#126,.T.);
#14356=EDGE_CURVE('',#11482,#11481,#9835,.T.);
#14357=EDGE_CURVE('',#11483,#11482,#127,.T.);
#14358=EDGE_CURVE('',#11484,#11483,#9836,.T.);
#14359=EDGE_CURVE('',#11484,#11485,#6170,.T.);
#14360=EDGE_CURVE('',#11485,#11485,#9837,.T.);
#14361=EDGE_CURVE('',#11486,#11484,#9838,.T.);
#14362=EDGE_CURVE('',#11487,#11486,#128,.T.);
#14363=EDGE_CURVE('',#11488,#11487,#9839,.T.);
#14364=EDGE_CURVE('',#11480,#11488,#129,.T.);
#14365=EDGE_CURVE('',#11489,#11489,#9840,.T.);
#14366=EDGE_CURVE('',#11489,#11490,#6171,.T.);
#14367=EDGE_CURVE('',#11490,#11490,#9841,.T.);
#14368=EDGE_CURVE('',#11491,#11492,#9842,.T.);
#14369=EDGE_CURVE('',#11493,#11491,#130,.T.);
#14370=EDGE_CURVE('',#11494,#11493,#9843,.T.);
#14371=EDGE_CURVE('',#11495,#11494,#131,.T.);
#14372=EDGE_CURVE('',#11496,#11495,#9844,.T.);
#14373=EDGE_CURVE('',#11496,#11497,#6172,.T.);
#14374=EDGE_CURVE('',#11497,#11497,#9845,.T.);
#14375=EDGE_CURVE('',#11498,#11496,#9846,.T.);
#14376=EDGE_CURVE('',#11499,#11498,#132,.T.);
#14377=EDGE_CURVE('',#11500,#11499,#9847,.T.);
#14378=EDGE_CURVE('',#11492,#11500,#133,.T.);
#14379=EDGE_CURVE('',#11501,#11501,#9848,.T.);
#14380=EDGE_CURVE('',#11501,#11502,#6173,.T.);
#14381=EDGE_CURVE('',#11502,#11502,#9849,.T.);
#14382=EDGE_CURVE('',#11503,#11504,#9850,.T.);
#14383=EDGE_CURVE('',#11505,#11503,#134,.T.);
#14384=EDGE_CURVE('',#11506,#11505,#9851,.T.);
#14385=EDGE_CURVE('',#11507,#11506,#135,.T.);
#14386=EDGE_CURVE('',#11508,#11507,#9852,.T.);
#14387=EDGE_CURVE('',#11508,#11509,#6174,.T.);
#14388=EDGE_CURVE('',#11509,#11509,#9853,.T.);
#14389=EDGE_CURVE('',#11510,#11508,#9854,.T.);
#14390=EDGE_CURVE('',#11511,#11510,#136,.T.);
#14391=EDGE_CURVE('',#11512,#11511,#9855,.T.);
#14392=EDGE_CURVE('',#11504,#11512,#137,.T.);
#14393=EDGE_CURVE('',#11513,#11513,#9856,.T.);
#14394=EDGE_CURVE('',#11513,#11514,#6175,.T.);
#14395=EDGE_CURVE('',#11514,#11514,#9857,.T.);
#14396=EDGE_CURVE('',#11515,#11516,#9858,.T.);
#14397=EDGE_CURVE('',#11517,#11515,#138,.T.);
#14398=EDGE_CURVE('',#11518,#11517,#9859,.T.);
#14399=EDGE_CURVE('',#11519,#11518,#139,.T.);
#14400=EDGE_CURVE('',#11520,#11519,#9860,.T.);
#14401=EDGE_CURVE('',#11520,#11521,#6176,.T.);
#14402=EDGE_CURVE('',#11521,#11521,#9861,.T.);
#14403=EDGE_CURVE('',#11522,#11520,#9862,.T.);
#14404=EDGE_CURVE('',#11523,#11522,#140,.T.);
#14405=EDGE_CURVE('',#11524,#11523,#9863,.T.);
#14406=EDGE_CURVE('',#11516,#11524,#141,.T.);
#14407=EDGE_CURVE('',#11525,#11525,#9864,.T.);
#14408=EDGE_CURVE('',#11525,#11526,#6177,.T.);
#14409=EDGE_CURVE('',#11526,#11526,#9865,.T.);
#14410=EDGE_CURVE('',#11527,#11528,#9866,.T.);
#14411=EDGE_CURVE('',#11529,#11527,#142,.T.);
#14412=EDGE_CURVE('',#11530,#11529,#9867,.T.);
#14413=EDGE_CURVE('',#11531,#11530,#143,.T.);
#14414=EDGE_CURVE('',#11532,#11531,#9868,.T.);
#14415=EDGE_CURVE('',#11532,#11533,#6178,.T.);
#14416=EDGE_CURVE('',#11533,#11533,#9869,.T.);
#14417=EDGE_CURVE('',#11534,#11532,#9870,.T.);
#14418=EDGE_CURVE('',#11535,#11534,#144,.T.);
#14419=EDGE_CURVE('',#11536,#11535,#9871,.T.);
#14420=EDGE_CURVE('',#11528,#11536,#145,.T.);
#14421=EDGE_CURVE('',#11537,#11447,#6179,.T.);
#14422=EDGE_CURVE('',#11538,#11446,#6180,.T.);
#14423=EDGE_CURVE('',#11537,#11538,#6181,.T.);
#14424=EDGE_CURVE('',#11443,#11459,#6182,.T.);
#14425=EDGE_CURVE('',#11444,#11462,#6183,.T.);
#14426=EDGE_CURVE('',#11452,#11463,#6184,.T.);
#14427=EDGE_CURVE('',#11445,#11458,#6185,.T.);
#14428=EDGE_CURVE('',#11457,#11470,#6186,.T.);
#14429=EDGE_CURVE('',#11469,#11482,#6187,.T.);
#14430=EDGE_CURVE('',#11481,#11494,#6188,.T.);
#14431=EDGE_CURVE('',#11493,#11506,#6189,.T.);
#14432=EDGE_CURVE('',#11505,#11518,#6190,.T.);
#14433=EDGE_CURVE('',#11517,#11530,#6191,.T.);
#14434=EDGE_CURVE('',#11529,#11539,#6192,.T.);
#14435=EDGE_CURVE('',#11540,#11539,#6193,.T.);
#14436=EDGE_CURVE('',#11541,#11540,#6194,.T.);
#14437=EDGE_CURVE('',#11541,#11538,#6195,.T.);
#14438=EDGE_CURVE('',#11542,#11451,#6196,.T.);
#14439=EDGE_CURVE('',#11542,#11543,#6197,.T.);
#14440=EDGE_CURVE('',#11543,#11544,#6198,.T.);
#14441=EDGE_CURVE('',#11545,#11544,#6199,.T.);
#14442=EDGE_CURVE('',#11536,#11545,#6200,.T.);
#14443=EDGE_CURVE('',#11524,#11535,#6201,.T.);
#14444=EDGE_CURVE('',#11512,#11523,#6202,.T.);
#14445=EDGE_CURVE('',#11500,#11511,#6203,.T.);
#14446=EDGE_CURVE('',#11488,#11499,#6204,.T.);
#14447=EDGE_CURVE('',#11476,#11487,#6205,.T.);
#14448=EDGE_CURVE('',#11464,#11475,#6206,.T.);
#14449=EDGE_CURVE('',#11455,#11471,#6207,.T.);
#14450=EDGE_CURVE('',#11456,#11474,#6208,.T.);
#14451=EDGE_CURVE('',#11467,#11483,#6209,.T.);
#14452=EDGE_CURVE('',#11468,#11486,#6210,.T.);
#14453=EDGE_CURVE('',#11480,#11498,#6211,.T.);
#14454=EDGE_CURVE('',#11479,#11495,#6212,.T.);
#14455=EDGE_CURVE('',#11491,#11507,#6213,.T.);
#14456=EDGE_CURVE('',#11492,#11510,#6214,.T.);
#14457=EDGE_CURVE('',#11503,#11519,#6215,.T.);
#14458=EDGE_CURVE('',#11504,#11522,#6216,.T.);
#14459=EDGE_CURVE('',#11515,#11531,#6217,.T.);
#14460=EDGE_CURVE('',#11516,#11534,#6218,.T.);
#14461=EDGE_CURVE('',#11527,#11546,#6219,.T.);
#14462=EDGE_CURVE('',#11528,#11547,#6220,.T.);
#14463=EDGE_CURVE('',#11547,#11546,#6221,.T.);
#14464=EDGE_CURVE('',#11545,#11547,#6222,.T.);
#14465=EDGE_CURVE('',#11548,#11541,#6223,.T.);
#14466=EDGE_CURVE('',#11549,#11548,#6224,.T.);
#14467=EDGE_CURVE('',#11549,#11550,#9872,.T.);
#14468=EDGE_CURVE('',#11551,#11550,#6225,.T.);
#14469=EDGE_CURVE('',#11551,#11552,#9873,.T.);
#14470=EDGE_CURVE('',#11553,#11552,#6226,.T.);
#14471=EDGE_CURVE('',#11553,#11554,#9874,.T.);
#14472=EDGE_CURVE('',#11555,#11554,#6227,.T.);
#14473=EDGE_CURVE('',#11555,#11556,#9875,.T.);
#14474=EDGE_CURVE('',#11556,#11557,#9876,.T.);
#14475=EDGE_CURVE('',#11557,#11558,#9877,.T.);
#14476=EDGE_CURVE('',#11559,#11558,#6228,.T.);
#14477=EDGE_CURVE('',#11559,#11560,#9878,.T.);
#14478=EDGE_CURVE('',#11561,#11560,#6229,.T.);
#14479=EDGE_CURVE('',#11561,#11562,#9879,.T.);
#14480=EDGE_CURVE('',#11563,#11562,#6230,.T.);
#14481=EDGE_CURVE('',#11563,#11564,#9880,.T.);
#14482=EDGE_CURVE('',#11564,#11565,#9881,.T.);
#14483=EDGE_CURVE('',#11565,#11566,#9882,.T.);
#14484=EDGE_CURVE('',#11567,#11566,#6231,.T.);
#14485=EDGE_CURVE('',#11568,#11567,#6232,.T.);
#14486=EDGE_CURVE('',#11568,#11569,#6233,.T.);
#14487=EDGE_CURVE('',#11569,#11570,#9883,.T.);
#14488=EDGE_CURVE('',#11571,#11570,#9884,.T.);
#14489=EDGE_CURVE('',#11571,#11572,#9885,.T.);
#14490=EDGE_CURVE('',#11572,#11573,#6234,.T.);
#14491=EDGE_CURVE('',#11573,#11574,#9886,.T.);
#14492=EDGE_CURVE('',#11574,#11575,#6235,.T.);
#14493=EDGE_CURVE('',#11575,#11576,#9887,.T.);
#14494=EDGE_CURVE('',#11576,#11577,#6236,.T.);
#14495=EDGE_CURVE('',#11577,#11578,#9888,.T.);
#14496=EDGE_CURVE('',#11579,#11578,#9889,.T.);
#14497=EDGE_CURVE('',#11579,#11580,#9890,.T.);
#14498=EDGE_CURVE('',#11580,#11581,#6237,.T.);
#14499=EDGE_CURVE('',#11581,#11582,#9891,.T.);
#14500=EDGE_CURVE('',#11582,#11583,#6238,.T.);
#14501=EDGE_CURVE('',#11583,#11584,#9892,.T.);
#14502=EDGE_CURVE('',#11584,#11585,#6239,.T.);
#14503=EDGE_CURVE('',#11585,#11586,#9893,.T.);
#14504=EDGE_CURVE('',#11586,#11587,#6240,.T.);
#14505=EDGE_CURVE('',#11587,#11543,#6241,.T.);
#14506=EDGE_CURVE('',#11542,#11588,#6242,.T.);
#14507=EDGE_CURVE('',#11588,#11537,#6243,.T.);
#14508=EDGE_CURVE('',#11546,#11539,#6244,.T.);
#14509=EDGE_CURVE('',#11589,#11544,#6245,.T.);
#14510=EDGE_CURVE('',#11590,#11589,#6246,.T.);
#14511=EDGE_CURVE('',#11590,#11591,#9894,.T.);
#14512=EDGE_CURVE('',#11592,#11591,#6247,.T.);
#14513=EDGE_CURVE('',#11592,#11593,#9895,.T.);
#14514=EDGE_CURVE('',#11594,#11593,#6248,.T.);
#14515=EDGE_CURVE('',#11594,#11595,#9896,.T.);
#14516=EDGE_CURVE('',#11596,#11595,#6249,.T.);
#14517=EDGE_CURVE('',#11596,#11597,#9897,.T.);
#14518=EDGE_CURVE('',#11597,#11598,#9898,.T.);
#14519=EDGE_CURVE('',#11598,#11599,#9899,.T.);
#14520=EDGE_CURVE('',#11600,#11599,#6250,.T.);
#14521=EDGE_CURVE('',#11600,#11601,#9900,.T.);
#14522=EDGE_CURVE('',#11602,#11601,#6251,.T.);
#14523=EDGE_CURVE('',#11602,#11603,#9901,.T.);
#14524=EDGE_CURVE('',#11604,#11603,#6252,.T.);
#14525=EDGE_CURVE('',#11604,#11605,#9902,.T.);
#14526=EDGE_CURVE('',#11605,#11606,#9903,.T.);
#14527=EDGE_CURVE('',#11606,#11607,#9904,.T.);
#14528=EDGE_CURVE('',#11608,#11607,#6253,.T.);
#14529=EDGE_CURVE('',#11608,#11609,#6254,.T.);
#14530=EDGE_CURVE('',#11609,#11610,#6255,.T.);
#14531=EDGE_CURVE('',#11610,#11611,#9905,.T.);
#14532=EDGE_CURVE('',#11612,#11611,#9906,.T.);
#14533=EDGE_CURVE('',#11612,#11613,#9907,.T.);
#14534=EDGE_CURVE('',#11613,#11614,#6256,.T.);
#14535=EDGE_CURVE('',#11614,#11615,#9908,.T.);
#14536=EDGE_CURVE('',#11615,#11616,#6257,.T.);
#14537=EDGE_CURVE('',#11616,#11617,#9909,.T.);
#14538=EDGE_CURVE('',#11617,#11618,#6258,.T.);
#14539=EDGE_CURVE('',#11618,#11619,#9910,.T.);
#14540=EDGE_CURVE('',#11620,#11619,#9911,.T.);
#14541=EDGE_CURVE('',#11620,#11621,#9912,.T.);
#14542=EDGE_CURVE('',#11621,#11622,#6259,.T.);
#14543=EDGE_CURVE('',#11622,#11623,#9913,.T.);
#14544=EDGE_CURVE('',#11623,#11624,#6260,.T.);
#14545=EDGE_CURVE('',#11624,#11625,#9914,.T.);
#14546=EDGE_CURVE('',#11625,#11626,#6261,.T.);
#14547=EDGE_CURVE('',#11626,#11627,#9915,.T.);
#14548=EDGE_CURVE('',#11627,#11628,#6262,.T.);
#14549=EDGE_CURVE('',#11628,#11540,#6263,.T.);
#14550=EDGE_CURVE('',#11595,#11581,#6264,.T.);
#14551=EDGE_CURVE('',#11580,#11596,#6265,.T.);
#14552=EDGE_CURVE('',#11576,#11600,#6266,.T.);
#14553=EDGE_CURVE('',#11599,#11577,#6267,.T.);
#14554=EDGE_CURVE('',#11572,#11604,#6268,.T.);
#14555=EDGE_CURVE('',#11603,#11573,#6269,.T.);
#14556=EDGE_CURVE('',#11607,#11569,#6270,.T.);
#14557=EDGE_CURVE('',#11568,#11608,#6271,.T.);
#14558=EDGE_CURVE('',#11554,#11622,#6272,.T.);
#14559=EDGE_CURVE('',#11621,#11555,#6273,.T.);
#14560=EDGE_CURVE('',#11613,#11563,#6274,.T.);
#14561=EDGE_CURVE('',#11562,#11614,#6275,.T.);
#14562=EDGE_CURVE('',#11567,#11609,#6276,.T.);
#14563=EDGE_CURVE('',#11548,#11628,#6277,.T.);
#14564=EDGE_CURVE('',#11627,#11549,#6278,.T.);
#14565=EDGE_CURVE('',#11550,#11626,#6279,.T.);
#14566=EDGE_CURVE('',#11625,#11551,#6280,.T.);
#14567=EDGE_CURVE('',#11552,#11624,#6281,.T.);
#14568=EDGE_CURVE('',#11623,#11553,#6282,.T.);
#14569=EDGE_CURVE('',#11617,#11559,#6283,.T.);
#14570=EDGE_CURVE('',#11558,#11618,#6284,.T.);
#14571=EDGE_CURVE('',#11615,#11561,#6285,.T.);
#14572=EDGE_CURVE('',#11560,#11616,#6286,.T.);
#14573=EDGE_CURVE('',#11566,#11610,#6287,.T.);
#14574=EDGE_CURVE('',#11564,#11612,#6288,.T.);
#14575=EDGE_CURVE('',#11611,#11565,#6289,.T.);
#14576=EDGE_CURVE('',#11619,#11557,#6290,.T.);
#14577=EDGE_CURVE('',#11556,#11620,#6291,.T.);
#14578=EDGE_CURVE('',#11574,#11602,#6292,.T.);
#14579=EDGE_CURVE('',#11601,#11575,#6293,.T.);
#14580=EDGE_CURVE('',#11593,#11583,#6294,.T.);
#14581=EDGE_CURVE('',#11582,#11594,#6295,.T.);
#14582=EDGE_CURVE('',#11591,#11585,#6296,.T.);
#14583=EDGE_CURVE('',#11584,#11592,#6297,.T.);
#14584=EDGE_CURVE('',#11586,#11590,#6298,.T.);
#14585=EDGE_CURVE('',#11587,#11589,#6299,.T.);
#14586=EDGE_CURVE('',#11605,#11571,#6300,.T.);
#14587=EDGE_CURVE('',#11570,#11606,#6301,.T.);
#14588=EDGE_CURVE('',#11578,#11598,#6302,.T.);
#14589=EDGE_CURVE('',#11597,#11579,#6303,.T.);
#14590=EDGE_CURVE('',#11588,#11450,#6304,.T.);
#19528=ORIENTED_EDGE('',*,*,#14309,.F.);
#19529=ORIENTED_EDGE('',*,*,#14310,.T.);
#19530=ORIENTED_EDGE('',*,*,#14311,.T.);
#19531=ORIENTED_EDGE('',*,*,#14310,.F.);
#19532=ORIENTED_EDGE('',*,*,#14312,.F.);
#19533=ORIENTED_EDGE('',*,*,#14313,.F.);
#19534=ORIENTED_EDGE('',*,*,#14314,.F.);
#19535=ORIENTED_EDGE('',*,*,#14315,.F.);
#19536=ORIENTED_EDGE('',*,*,#14316,.F.);
#19537=ORIENTED_EDGE('',*,*,#14317,.T.);
#19538=ORIENTED_EDGE('',*,*,#14318,.T.);
#19539=ORIENTED_EDGE('',*,*,#14317,.F.);
#19540=ORIENTED_EDGE('',*,*,#14319,.F.);
#19541=ORIENTED_EDGE('',*,*,#14320,.F.);
#19542=ORIENTED_EDGE('',*,*,#14321,.F.);
#19543=ORIENTED_EDGE('',*,*,#14322,.F.);
#19544=ORIENTED_EDGE('',*,*,#14323,.F.);
#19545=ORIENTED_EDGE('',*,*,#14324,.T.);
#19546=ORIENTED_EDGE('',*,*,#14325,.T.);
#19547=ORIENTED_EDGE('',*,*,#14324,.F.);
#19548=ORIENTED_EDGE('',*,*,#14326,.F.);
#19549=ORIENTED_EDGE('',*,*,#14327,.F.);
#19550=ORIENTED_EDGE('',*,*,#14328,.F.);
#19551=ORIENTED_EDGE('',*,*,#14329,.F.);
#19552=ORIENTED_EDGE('',*,*,#14330,.F.);
#19553=ORIENTED_EDGE('',*,*,#14331,.T.);
#19554=ORIENTED_EDGE('',*,*,#14332,.T.);
#19555=ORIENTED_EDGE('',*,*,#14331,.F.);
#19556=ORIENTED_EDGE('',*,*,#14333,.F.);
#19557=ORIENTED_EDGE('',*,*,#14334,.F.);
#19558=ORIENTED_EDGE('',*,*,#14335,.F.);
#19559=ORIENTED_EDGE('',*,*,#14336,.F.);
#19560=ORIENTED_EDGE('',*,*,#14337,.F.);
#19561=ORIENTED_EDGE('',*,*,#14338,.T.);
#19562=ORIENTED_EDGE('',*,*,#14339,.T.);
#19563=ORIENTED_EDGE('',*,*,#14338,.F.);
#19564=ORIENTED_EDGE('',*,*,#14340,.F.);
#19565=ORIENTED_EDGE('',*,*,#14341,.F.);
#19566=ORIENTED_EDGE('',*,*,#14342,.F.);
#19567=ORIENTED_EDGE('',*,*,#14343,.F.);
#19568=ORIENTED_EDGE('',*,*,#14344,.F.);
#19569=ORIENTED_EDGE('',*,*,#14345,.T.);
#19570=ORIENTED_EDGE('',*,*,#14346,.T.);
#19571=ORIENTED_EDGE('',*,*,#14345,.F.);
#19572=ORIENTED_EDGE('',*,*,#14347,.F.);
#19573=ORIENTED_EDGE('',*,*,#14348,.F.);
#19574=ORIENTED_EDGE('',*,*,#14349,.F.);
#19575=ORIENTED_EDGE('',*,*,#14350,.F.);
#19576=ORIENTED_EDGE('',*,*,#14351,.F.);
#19577=ORIENTED_EDGE('',*,*,#14352,.T.);
#19578=ORIENTED_EDGE('',*,*,#14353,.T.);
#19579=ORIENTED_EDGE('',*,*,#14352,.F.);
#19580=ORIENTED_EDGE('',*,*,#14354,.F.);
#19581=ORIENTED_EDGE('',*,*,#14355,.F.);
#19582=ORIENTED_EDGE('',*,*,#14356,.F.);
#19583=ORIENTED_EDGE('',*,*,#14357,.F.);
#19584=ORIENTED_EDGE('',*,*,#14358,.F.);
#19585=ORIENTED_EDGE('',*,*,#14359,.T.);
#19586=ORIENTED_EDGE('',*,*,#14360,.T.);
#19587=ORIENTED_EDGE('',*,*,#14359,.F.);
#19588=ORIENTED_EDGE('',*,*,#14361,.F.);
#19589=ORIENTED_EDGE('',*,*,#14362,.F.);
#19590=ORIENTED_EDGE('',*,*,#14363,.F.);
#19591=ORIENTED_EDGE('',*,*,#14364,.F.);
#19592=ORIENTED_EDGE('',*,*,#14365,.F.);
#19593=ORIENTED_EDGE('',*,*,#14366,.T.);
#19594=ORIENTED_EDGE('',*,*,#14367,.T.);
#19595=ORIENTED_EDGE('',*,*,#14366,.F.);
#19596=ORIENTED_EDGE('',*,*,#14368,.F.);
#19597=ORIENTED_EDGE('',*,*,#14369,.F.);
#19598=ORIENTED_EDGE('',*,*,#14370,.F.);
#19599=ORIENTED_EDGE('',*,*,#14371,.F.);
#19600=ORIENTED_EDGE('',*,*,#14372,.F.);
#19601=ORIENTED_EDGE('',*,*,#14373,.T.);
#19602=ORIENTED_EDGE('',*,*,#14374,.T.);
#19603=ORIENTED_EDGE('',*,*,#14373,.F.);
#19604=ORIENTED_EDGE('',*,*,#14375,.F.);
#19605=ORIENTED_EDGE('',*,*,#14376,.F.);
#19606=ORIENTED_EDGE('',*,*,#14377,.F.);
#19607=ORIENTED_EDGE('',*,*,#14378,.F.);
#19608=ORIENTED_EDGE('',*,*,#14379,.F.);
#19609=ORIENTED_EDGE('',*,*,#14380,.T.);
#19610=ORIENTED_EDGE('',*,*,#14381,.T.);
#19611=ORIENTED_EDGE('',*,*,#14380,.F.);
#19612=ORIENTED_EDGE('',*,*,#14382,.F.);
#19613=ORIENTED_EDGE('',*,*,#14383,.F.);
#19614=ORIENTED_EDGE('',*,*,#14384,.F.);
#19615=ORIENTED_EDGE('',*,*,#14385,.F.);
#19616=ORIENTED_EDGE('',*,*,#14386,.F.);
#19617=ORIENTED_EDGE('',*,*,#14387,.T.);
#19618=ORIENTED_EDGE('',*,*,#14388,.T.);
#19619=ORIENTED_EDGE('',*,*,#14387,.F.);
#19620=ORIENTED_EDGE('',*,*,#14389,.F.);
#19621=ORIENTED_EDGE('',*,*,#14390,.F.);
#19622=ORIENTED_EDGE('',*,*,#14391,.F.);
#19623=ORIENTED_EDGE('',*,*,#14392,.F.);
#19624=ORIENTED_EDGE('',*,*,#14393,.F.);
#19625=ORIENTED_EDGE('',*,*,#14394,.T.);
#19626=ORIENTED_EDGE('',*,*,#14395,.T.);
#19627=ORIENTED_EDGE('',*,*,#14394,.F.);
#19628=ORIENTED_EDGE('',*,*,#14396,.F.);
#19629=ORIENTED_EDGE('',*,*,#14397,.F.);
#19630=ORIENTED_EDGE('',*,*,#14398,.F.);
#19631=ORIENTED_EDGE('',*,*,#14399,.F.);
#19632=ORIENTED_EDGE('',*,*,#14400,.F.);
#19633=ORIENTED_EDGE('',*,*,#14401,.T.);
#19634=ORIENTED_EDGE('',*,*,#14402,.T.);
#19635=ORIENTED_EDGE('',*,*,#14401,.F.);
#19636=ORIENTED_EDGE('',*,*,#14403,.F.);
#19637=ORIENTED_EDGE('',*,*,#14404,.F.);
#19638=ORIENTED_EDGE('',*,*,#14405,.F.);
#19639=ORIENTED_EDGE('',*,*,#14406,.F.);
#19640=ORIENTED_EDGE('',*,*,#14407,.F.);
#19641=ORIENTED_EDGE('',*,*,#14408,.T.);
#19642=ORIENTED_EDGE('',*,*,#14409,.T.);
#19643=ORIENTED_EDGE('',*,*,#14408,.F.);
#19644=ORIENTED_EDGE('',*,*,#14410,.F.);
#19645=ORIENTED_EDGE('',*,*,#14411,.F.);
#19646=ORIENTED_EDGE('',*,*,#14412,.F.);
#19647=ORIENTED_EDGE('',*,*,#14413,.F.);
#19648=ORIENTED_EDGE('',*,*,#14414,.F.);
#19649=ORIENTED_EDGE('',*,*,#14415,.T.);
#19650=ORIENTED_EDGE('',*,*,#14416,.T.);
#19651=ORIENTED_EDGE('',*,*,#14415,.F.);
#19652=ORIENTED_EDGE('',*,*,#14417,.F.);
#19653=ORIENTED_EDGE('',*,*,#14418,.F.);
#19654=ORIENTED_EDGE('',*,*,#14419,.F.);
#19655=ORIENTED_EDGE('',*,*,#14420,.F.);
#19656=ORIENTED_EDGE('',*,*,#14421,.T.);
#19657=ORIENTED_EDGE('',*,*,#14315,.T.);
#19658=ORIENTED_EDGE('',*,*,#14422,.F.);
#19659=ORIENTED_EDGE('',*,*,#14423,.F.);
#19660=ORIENTED_EDGE('',*,*,#14424,.F.);
#19661=ORIENTED_EDGE('',*,*,#14312,.T.);
#19662=ORIENTED_EDGE('',*,*,#14425,.T.);
#19663=ORIENTED_EDGE('',*,*,#14333,.T.);
#19664=ORIENTED_EDGE('',*,*,#14330,.T.);
#19665=ORIENTED_EDGE('',*,*,#14425,.F.);
#19666=ORIENTED_EDGE('',*,*,#14322,.T.);
#19667=ORIENTED_EDGE('',*,*,#14426,.T.);
#19668=ORIENTED_EDGE('',*,*,#14334,.T.);
#19669=ORIENTED_EDGE('',*,*,#14422,.T.);
#19670=ORIENTED_EDGE('',*,*,#14314,.T.);
#19671=ORIENTED_EDGE('',*,*,#14427,.T.);
#19672=ORIENTED_EDGE('',*,*,#14328,.T.);
#19673=ORIENTED_EDGE('',*,*,#14428,.T.);
#19674=ORIENTED_EDGE('',*,*,#14342,.T.);
#19675=ORIENTED_EDGE('',*,*,#14429,.T.);
#19676=ORIENTED_EDGE('',*,*,#14356,.T.);
#19677=ORIENTED_EDGE('',*,*,#14430,.T.);
#19678=ORIENTED_EDGE('',*,*,#14370,.T.);
#19679=ORIENTED_EDGE('',*,*,#14431,.T.);
#19680=ORIENTED_EDGE('',*,*,#14384,.T.);
#19681=ORIENTED_EDGE('',*,*,#14432,.T.);
#19682=ORIENTED_EDGE('',*,*,#14398,.T.);
#19683=ORIENTED_EDGE('',*,*,#14433,.T.);
#19684=ORIENTED_EDGE('',*,*,#14412,.T.);
#19685=ORIENTED_EDGE('',*,*,#14434,.T.);
#19686=ORIENTED_EDGE('',*,*,#14435,.F.);
#19687=ORIENTED_EDGE('',*,*,#14436,.F.);
#19688=ORIENTED_EDGE('',*,*,#14437,.T.);
#19689=ORIENTED_EDGE('',*,*,#14426,.F.);
#19690=ORIENTED_EDGE('',*,*,#14321,.T.);
#19691=ORIENTED_EDGE('',*,*,#14438,.F.);
#19692=ORIENTED_EDGE('',*,*,#14439,.T.);
#19693=ORIENTED_EDGE('',*,*,#14440,.T.);
#19694=ORIENTED_EDGE('',*,*,#14441,.F.);
#19695=ORIENTED_EDGE('',*,*,#14442,.F.);
#19696=ORIENTED_EDGE('',*,*,#14419,.T.);
#19697=ORIENTED_EDGE('',*,*,#14443,.F.);
#19698=ORIENTED_EDGE('',*,*,#14405,.T.);
#19699=ORIENTED_EDGE('',*,*,#14444,.F.);
#19700=ORIENTED_EDGE('',*,*,#14391,.T.);
#19701=ORIENTED_EDGE('',*,*,#14445,.F.);
#19702=ORIENTED_EDGE('',*,*,#14377,.T.);
#19703=ORIENTED_EDGE('',*,*,#14446,.F.);
#19704=ORIENTED_EDGE('',*,*,#14363,.T.);
#19705=ORIENTED_EDGE('',*,*,#14447,.F.);
#19706=ORIENTED_EDGE('',*,*,#14349,.T.);
#19707=ORIENTED_EDGE('',*,*,#14448,.F.);
#19708=ORIENTED_EDGE('',*,*,#14335,.T.);
#19709=ORIENTED_EDGE('',*,*,#14427,.F.);
#19710=ORIENTED_EDGE('',*,*,#14313,.T.);
#19711=ORIENTED_EDGE('',*,*,#14424,.T.);
#19712=ORIENTED_EDGE('',*,*,#14329,.T.);
#19713=ORIENTED_EDGE('',*,*,#14449,.F.);
#19714=ORIENTED_EDGE('',*,*,#14326,.T.);
#19715=ORIENTED_EDGE('',*,*,#14450,.T.);
#19716=ORIENTED_EDGE('',*,*,#14347,.T.);
#19717=ORIENTED_EDGE('',*,*,#14344,.T.);
#19718=ORIENTED_EDGE('',*,*,#14450,.F.);
#19719=ORIENTED_EDGE('',*,*,#14336,.T.);
#19720=ORIENTED_EDGE('',*,*,#14448,.T.);
#19721=ORIENTED_EDGE('',*,*,#14348,.T.);
#19722=ORIENTED_EDGE('',*,*,#14428,.F.);
#19723=ORIENTED_EDGE('',*,*,#14327,.T.);
#19724=ORIENTED_EDGE('',*,*,#14449,.T.);
#19725=ORIENTED_EDGE('',*,*,#14343,.T.);
#19726=ORIENTED_EDGE('',*,*,#14451,.F.);
#19727=ORIENTED_EDGE('',*,*,#14340,.T.);
#19728=ORIENTED_EDGE('',*,*,#14452,.T.);
#19729=ORIENTED_EDGE('',*,*,#14361,.T.);
#19730=ORIENTED_EDGE('',*,*,#14358,.T.);
#19731=ORIENTED_EDGE('',*,*,#14452,.F.);
#19732=ORIENTED_EDGE('',*,*,#14350,.T.);
#19733=ORIENTED_EDGE('',*,*,#14447,.T.);
#19734=ORIENTED_EDGE('',*,*,#14362,.T.);
#19735=ORIENTED_EDGE('',*,*,#14429,.F.);
#19736=ORIENTED_EDGE('',*,*,#14341,.T.);
#19737=ORIENTED_EDGE('',*,*,#14451,.T.);
#19738=ORIENTED_EDGE('',*,*,#14357,.T.);
#19739=ORIENTED_EDGE('',*,*,#14453,.F.);
#19740=ORIENTED_EDGE('',*,*,#14364,.T.);
#19741=ORIENTED_EDGE('',*,*,#14446,.T.);
#19742=ORIENTED_EDGE('',*,*,#14376,.T.);
#19743=ORIENTED_EDGE('',*,*,#14454,.F.);
#19744=ORIENTED_EDGE('',*,*,#14354,.T.);
#19745=ORIENTED_EDGE('',*,*,#14453,.T.);
#19746=ORIENTED_EDGE('',*,*,#14375,.T.);
#19747=ORIENTED_EDGE('',*,*,#14372,.T.);
#19748=ORIENTED_EDGE('',*,*,#14430,.F.);
#19749=ORIENTED_EDGE('',*,*,#14355,.T.);
#19750=ORIENTED_EDGE('',*,*,#14454,.T.);
#19751=ORIENTED_EDGE('',*,*,#14371,.T.);
#19752=ORIENTED_EDGE('',*,*,#14455,.F.);
#19753=ORIENTED_EDGE('',*,*,#14368,.T.);
#19754=ORIENTED_EDGE('',*,*,#14456,.T.);
#19755=ORIENTED_EDGE('',*,*,#14389,.T.);
#19756=ORIENTED_EDGE('',*,*,#14386,.T.);
#19757=ORIENTED_EDGE('',*,*,#14456,.F.);
#19758=ORIENTED_EDGE('',*,*,#14378,.T.);
#19759=ORIENTED_EDGE('',*,*,#14445,.T.);
#19760=ORIENTED_EDGE('',*,*,#14390,.T.);
#19761=ORIENTED_EDGE('',*,*,#14431,.F.);
#19762=ORIENTED_EDGE('',*,*,#14369,.T.);
#19763=ORIENTED_EDGE('',*,*,#14455,.T.);
#19764=ORIENTED_EDGE('',*,*,#14385,.T.);
#19765=ORIENTED_EDGE('',*,*,#14457,.F.);
#19766=ORIENTED_EDGE('',*,*,#14382,.T.);
#19767=ORIENTED_EDGE('',*,*,#14458,.T.);
#19768=ORIENTED_EDGE('',*,*,#14403,.T.);
#19769=ORIENTED_EDGE('',*,*,#14400,.T.);
#19770=ORIENTED_EDGE('',*,*,#14458,.F.);
#19771=ORIENTED_EDGE('',*,*,#14392,.T.);
#19772=ORIENTED_EDGE('',*,*,#14444,.T.);
#19773=ORIENTED_EDGE('',*,*,#14404,.T.);
#19774=ORIENTED_EDGE('',*,*,#14432,.F.);
#19775=ORIENTED_EDGE('',*,*,#14383,.T.);
#19776=ORIENTED_EDGE('',*,*,#14457,.T.);
#19777=ORIENTED_EDGE('',*,*,#14399,.T.);
#19778=ORIENTED_EDGE('',*,*,#14459,.F.);
#19779=ORIENTED_EDGE('',*,*,#14396,.T.);
#19780=ORIENTED_EDGE('',*,*,#14460,.T.);
#19781=ORIENTED_EDGE('',*,*,#14417,.T.);
#19782=ORIENTED_EDGE('',*,*,#14414,.T.);
#19783=ORIENTED_EDGE('',*,*,#14460,.F.);
#19784=ORIENTED_EDGE('',*,*,#14406,.T.);
#19785=ORIENTED_EDGE('',*,*,#14443,.T.);
#19786=ORIENTED_EDGE('',*,*,#14418,.T.);
#19787=ORIENTED_EDGE('',*,*,#14433,.F.);
#19788=ORIENTED_EDGE('',*,*,#14397,.T.);
#19789=ORIENTED_EDGE('',*,*,#14459,.T.);
#19790=ORIENTED_EDGE('',*,*,#14413,.T.);
#19791=ORIENTED_EDGE('',*,*,#14461,.F.);
#19792=ORIENTED_EDGE('',*,*,#14410,.T.);
#19793=ORIENTED_EDGE('',*,*,#14462,.T.);
#19794=ORIENTED_EDGE('',*,*,#14463,.T.);
#19795=ORIENTED_EDGE('',*,*,#14462,.F.);
#19796=ORIENTED_EDGE('',*,*,#14420,.T.);
#19797=ORIENTED_EDGE('',*,*,#14442,.T.);
#19798=ORIENTED_EDGE('',*,*,#14464,.T.);
#19799=ORIENTED_EDGE('',*,*,#14423,.T.);
#19800=ORIENTED_EDGE('',*,*,#14437,.F.);
#19801=ORIENTED_EDGE('',*,*,#14465,.F.);
#19802=ORIENTED_EDGE('',*,*,#14466,.F.);
#19803=ORIENTED_EDGE('',*,*,#14467,.T.);
#19804=ORIENTED_EDGE('',*,*,#14468,.F.);
#19805=ORIENTED_EDGE('',*,*,#14469,.T.);
#19806=ORIENTED_EDGE('',*,*,#14470,.F.);
#19807=ORIENTED_EDGE('',*,*,#14471,.T.);
#19808=ORIENTED_EDGE('',*,*,#14472,.F.);
#19809=ORIENTED_EDGE('',*,*,#14473,.T.);
#19810=ORIENTED_EDGE('',*,*,#14474,.T.);
#19811=ORIENTED_EDGE('',*,*,#14475,.T.);
#19812=ORIENTED_EDGE('',*,*,#14476,.F.);
#19813=ORIENTED_EDGE('',*,*,#14477,.T.);
#19814=ORIENTED_EDGE('',*,*,#14478,.F.);
#19815=ORIENTED_EDGE('',*,*,#14479,.T.);
#19816=ORIENTED_EDGE('',*,*,#14480,.F.);
#19817=ORIENTED_EDGE('',*,*,#14481,.T.);
#19818=ORIENTED_EDGE('',*,*,#14482,.T.);
#19819=ORIENTED_EDGE('',*,*,#14483,.T.);
#19820=ORIENTED_EDGE('',*,*,#14484,.F.);
#19821=ORIENTED_EDGE('',*,*,#14485,.F.);
#19822=ORIENTED_EDGE('',*,*,#14486,.T.);
#19823=ORIENTED_EDGE('',*,*,#14487,.T.);
#19824=ORIENTED_EDGE('',*,*,#14488,.F.);
#19825=ORIENTED_EDGE('',*,*,#14489,.T.);
#19826=ORIENTED_EDGE('',*,*,#14490,.T.);
#19827=ORIENTED_EDGE('',*,*,#14491,.T.);
#19828=ORIENTED_EDGE('',*,*,#14492,.T.);
#19829=ORIENTED_EDGE('',*,*,#14493,.T.);
#19830=ORIENTED_EDGE('',*,*,#14494,.T.);
#19831=ORIENTED_EDGE('',*,*,#14495,.T.);
#19832=ORIENTED_EDGE('',*,*,#14496,.F.);
#19833=ORIENTED_EDGE('',*,*,#14497,.T.);
#19834=ORIENTED_EDGE('',*,*,#14498,.T.);
#19835=ORIENTED_EDGE('',*,*,#14499,.T.);
#19836=ORIENTED_EDGE('',*,*,#14500,.T.);
#19837=ORIENTED_EDGE('',*,*,#14501,.T.);
#19838=ORIENTED_EDGE('',*,*,#14502,.T.);
#19839=ORIENTED_EDGE('',*,*,#14503,.T.);
#19840=ORIENTED_EDGE('',*,*,#14504,.T.);
#19841=ORIENTED_EDGE('',*,*,#14505,.T.);
#19842=ORIENTED_EDGE('',*,*,#14439,.F.);
#19843=ORIENTED_EDGE('',*,*,#14506,.T.);
#19844=ORIENTED_EDGE('',*,*,#14507,.T.);
#19845=ORIENTED_EDGE('',*,*,#14435,.T.);
#19846=ORIENTED_EDGE('',*,*,#14508,.F.);
#19847=ORIENTED_EDGE('',*,*,#14463,.F.);
#19848=ORIENTED_EDGE('',*,*,#14464,.F.);
#19849=ORIENTED_EDGE('',*,*,#14441,.T.);
#19850=ORIENTED_EDGE('',*,*,#14509,.F.);
#19851=ORIENTED_EDGE('',*,*,#14510,.F.);
#19852=ORIENTED_EDGE('',*,*,#14511,.T.);
#19853=ORIENTED_EDGE('',*,*,#14512,.F.);
#19854=ORIENTED_EDGE('',*,*,#14513,.T.);
#19855=ORIENTED_EDGE('',*,*,#14514,.F.);
#19856=ORIENTED_EDGE('',*,*,#14515,.T.);
#19857=ORIENTED_EDGE('',*,*,#14516,.F.);
#19858=ORIENTED_EDGE('',*,*,#14517,.T.);
#19859=ORIENTED_EDGE('',*,*,#14518,.T.);
#19860=ORIENTED_EDGE('',*,*,#14519,.T.);
#19861=ORIENTED_EDGE('',*,*,#14520,.F.);
#19862=ORIENTED_EDGE('',*,*,#14521,.T.);
#19863=ORIENTED_EDGE('',*,*,#14522,.F.);
#19864=ORIENTED_EDGE('',*,*,#14523,.T.);
#19865=ORIENTED_EDGE('',*,*,#14524,.F.);
#19866=ORIENTED_EDGE('',*,*,#14525,.T.);
#19867=ORIENTED_EDGE('',*,*,#14526,.T.);
#19868=ORIENTED_EDGE('',*,*,#14527,.T.);
#19869=ORIENTED_EDGE('',*,*,#14528,.F.);
#19870=ORIENTED_EDGE('',*,*,#14529,.T.);
#19871=ORIENTED_EDGE('',*,*,#14530,.T.);
#19872=ORIENTED_EDGE('',*,*,#14531,.T.);
#19873=ORIENTED_EDGE('',*,*,#14532,.F.);
#19874=ORIENTED_EDGE('',*,*,#14533,.T.);
#19875=ORIENTED_EDGE('',*,*,#14534,.T.);
#19876=ORIENTED_EDGE('',*,*,#14535,.T.);
#19877=ORIENTED_EDGE('',*,*,#14536,.T.);
#19878=ORIENTED_EDGE('',*,*,#14537,.T.);
#19879=ORIENTED_EDGE('',*,*,#14538,.T.);
#19880=ORIENTED_EDGE('',*,*,#14539,.T.);
#19881=ORIENTED_EDGE('',*,*,#14540,.F.);
#19882=ORIENTED_EDGE('',*,*,#14541,.T.);
#19883=ORIENTED_EDGE('',*,*,#14542,.T.);
#19884=ORIENTED_EDGE('',*,*,#14543,.T.);
#19885=ORIENTED_EDGE('',*,*,#14544,.T.);
#19886=ORIENTED_EDGE('',*,*,#14545,.T.);
#19887=ORIENTED_EDGE('',*,*,#14546,.T.);
#19888=ORIENTED_EDGE('',*,*,#14547,.T.);
#19889=ORIENTED_EDGE('',*,*,#14548,.T.);
#19890=ORIENTED_EDGE('',*,*,#14549,.T.);
#19891=ORIENTED_EDGE('',*,*,#14516,.T.);
#19892=ORIENTED_EDGE('',*,*,#14550,.T.);
#19893=ORIENTED_EDGE('',*,*,#14498,.F.);
#19894=ORIENTED_EDGE('',*,*,#14551,.T.);
#19895=ORIENTED_EDGE('',*,*,#14494,.F.);
#19896=ORIENTED_EDGE('',*,*,#14552,.T.);
#19897=ORIENTED_EDGE('',*,*,#14520,.T.);
#19898=ORIENTED_EDGE('',*,*,#14553,.T.);
#19899=ORIENTED_EDGE('',*,*,#14490,.F.);
#19900=ORIENTED_EDGE('',*,*,#14554,.T.);
#19901=ORIENTED_EDGE('',*,*,#14524,.T.);
#19902=ORIENTED_EDGE('',*,*,#14555,.T.);
#19903=ORIENTED_EDGE('',*,*,#14528,.T.);
#19904=ORIENTED_EDGE('',*,*,#14556,.T.);
#19905=ORIENTED_EDGE('',*,*,#14486,.F.);
#19906=ORIENTED_EDGE('',*,*,#14557,.T.);
#19907=ORIENTED_EDGE('',*,*,#14472,.T.);
#19908=ORIENTED_EDGE('',*,*,#14558,.T.);
#19909=ORIENTED_EDGE('',*,*,#14542,.F.);
#19910=ORIENTED_EDGE('',*,*,#14559,.T.);
#19911=ORIENTED_EDGE('',*,*,#14534,.F.);
#19912=ORIENTED_EDGE('',*,*,#14560,.T.);
#19913=ORIENTED_EDGE('',*,*,#14480,.T.);
#19914=ORIENTED_EDGE('',*,*,#14561,.T.);
#19915=ORIENTED_EDGE('',*,*,#14529,.F.);
#19916=ORIENTED_EDGE('',*,*,#14557,.F.);
#19917=ORIENTED_EDGE('',*,*,#14485,.T.);
#19918=ORIENTED_EDGE('',*,*,#14562,.T.);
#19919=ORIENTED_EDGE('',*,*,#14311,.F.);
#19920=ORIENTED_EDGE('',*,*,#14325,.F.);
#19921=ORIENTED_EDGE('',*,*,#14339,.F.);
#19922=ORIENTED_EDGE('',*,*,#14353,.F.);
#19923=ORIENTED_EDGE('',*,*,#14367,.F.);
#19924=ORIENTED_EDGE('',*,*,#14381,.F.);
#19925=ORIENTED_EDGE('',*,*,#14395,.F.);
#19926=ORIENTED_EDGE('',*,*,#14409,.F.);
#19927=ORIENTED_EDGE('',*,*,#14549,.F.);
#19928=ORIENTED_EDGE('',*,*,#14563,.F.);
#19929=ORIENTED_EDGE('',*,*,#14465,.T.);
#19930=ORIENTED_EDGE('',*,*,#14436,.T.);
#19931=ORIENTED_EDGE('',*,*,#14548,.F.);
#19932=ORIENTED_EDGE('',*,*,#14564,.T.);
#19933=ORIENTED_EDGE('',*,*,#14466,.T.);
#19934=ORIENTED_EDGE('',*,*,#14563,.T.);
#19935=ORIENTED_EDGE('',*,*,#14468,.T.);
#19936=ORIENTED_EDGE('',*,*,#14565,.T.);
#19937=ORIENTED_EDGE('',*,*,#14546,.F.);
#19938=ORIENTED_EDGE('',*,*,#14566,.T.);
#19939=ORIENTED_EDGE('',*,*,#14470,.T.);
#19940=ORIENTED_EDGE('',*,*,#14567,.T.);
#19941=ORIENTED_EDGE('',*,*,#14544,.F.);
#19942=ORIENTED_EDGE('',*,*,#14568,.T.);
#19943=ORIENTED_EDGE('',*,*,#14538,.F.);
#19944=ORIENTED_EDGE('',*,*,#14569,.T.);
#19945=ORIENTED_EDGE('',*,*,#14476,.T.);
#19946=ORIENTED_EDGE('',*,*,#14570,.T.);
#19947=ORIENTED_EDGE('',*,*,#14536,.F.);
#19948=ORIENTED_EDGE('',*,*,#14571,.T.);
#19949=ORIENTED_EDGE('',*,*,#14478,.T.);
#19950=ORIENTED_EDGE('',*,*,#14572,.T.);
#19951=ORIENTED_EDGE('',*,*,#14484,.T.);
#19952=ORIENTED_EDGE('',*,*,#14573,.T.);
#19953=ORIENTED_EDGE('',*,*,#14530,.F.);
#19954=ORIENTED_EDGE('',*,*,#14562,.F.);
#19955=ORIENTED_EDGE('',*,*,#14482,.F.);
#19956=ORIENTED_EDGE('',*,*,#14574,.T.);
#19957=ORIENTED_EDGE('',*,*,#14532,.T.);
#19958=ORIENTED_EDGE('',*,*,#14575,.T.);
#19959=ORIENTED_EDGE('',*,*,#14540,.T.);
#19960=ORIENTED_EDGE('',*,*,#14576,.T.);
#19961=ORIENTED_EDGE('',*,*,#14474,.F.);
#19962=ORIENTED_EDGE('',*,*,#14577,.T.);
#19963=ORIENTED_EDGE('',*,*,#14481,.F.);
#19964=ORIENTED_EDGE('',*,*,#14560,.F.);
#19965=ORIENTED_EDGE('',*,*,#14533,.F.);
#19966=ORIENTED_EDGE('',*,*,#14574,.F.);
#19967=ORIENTED_EDGE('',*,*,#14479,.F.);
#19968=ORIENTED_EDGE('',*,*,#14571,.F.);
#19969=ORIENTED_EDGE('',*,*,#14535,.F.);
#19970=ORIENTED_EDGE('',*,*,#14561,.F.);
#19971=ORIENTED_EDGE('',*,*,#14477,.F.);
#19972=ORIENTED_EDGE('',*,*,#14569,.F.);
#19973=ORIENTED_EDGE('',*,*,#14537,.F.);
#19974=ORIENTED_EDGE('',*,*,#14572,.F.);
#19975=ORIENTED_EDGE('',*,*,#14539,.F.);
#19976=ORIENTED_EDGE('',*,*,#14570,.F.);
#19977=ORIENTED_EDGE('',*,*,#14475,.F.);
#19978=ORIENTED_EDGE('',*,*,#14576,.F.);
#19979=ORIENTED_EDGE('',*,*,#14469,.F.);
#19980=ORIENTED_EDGE('',*,*,#14566,.F.);
#19981=ORIENTED_EDGE('',*,*,#14545,.F.);
#19982=ORIENTED_EDGE('',*,*,#14567,.F.);
#19983=ORIENTED_EDGE('',*,*,#14471,.F.);
#19984=ORIENTED_EDGE('',*,*,#14568,.F.);
#19985=ORIENTED_EDGE('',*,*,#14543,.F.);
#19986=ORIENTED_EDGE('',*,*,#14558,.F.);
#19987=ORIENTED_EDGE('',*,*,#14473,.F.);
#19988=ORIENTED_EDGE('',*,*,#14559,.F.);
#19989=ORIENTED_EDGE('',*,*,#14541,.F.);
#19990=ORIENTED_EDGE('',*,*,#14577,.F.);
#19991=ORIENTED_EDGE('',*,*,#14531,.F.);
#19992=ORIENTED_EDGE('',*,*,#14573,.F.);
#19993=ORIENTED_EDGE('',*,*,#14483,.F.);
#19994=ORIENTED_EDGE('',*,*,#14575,.F.);
#19995=ORIENTED_EDGE('',*,*,#14467,.F.);
#19996=ORIENTED_EDGE('',*,*,#14564,.F.);
#19997=ORIENTED_EDGE('',*,*,#14547,.F.);
#19998=ORIENTED_EDGE('',*,*,#14565,.F.);
#19999=ORIENTED_EDGE('',*,*,#14492,.F.);
#20000=ORIENTED_EDGE('',*,*,#14578,.T.);
#20001=ORIENTED_EDGE('',*,*,#14522,.T.);
#20002=ORIENTED_EDGE('',*,*,#14579,.T.);
#20003=ORIENTED_EDGE('',*,*,#14514,.T.);
#20004=ORIENTED_EDGE('',*,*,#14580,.T.);
#20005=ORIENTED_EDGE('',*,*,#14500,.F.);
#20006=ORIENTED_EDGE('',*,*,#14581,.T.);
#20007=ORIENTED_EDGE('',*,*,#14512,.T.);
#20008=ORIENTED_EDGE('',*,*,#14582,.T.);
#20009=ORIENTED_EDGE('',*,*,#14502,.F.);
#20010=ORIENTED_EDGE('',*,*,#14583,.T.);
#20011=ORIENTED_EDGE('',*,*,#14504,.F.);
#20012=ORIENTED_EDGE('',*,*,#14584,.T.);
#20013=ORIENTED_EDGE('',*,*,#14510,.T.);
#20014=ORIENTED_EDGE('',*,*,#14585,.F.);
#20015=ORIENTED_EDGE('',*,*,#14509,.T.);
#20016=ORIENTED_EDGE('',*,*,#14440,.F.);
#20017=ORIENTED_EDGE('',*,*,#14505,.F.);
#20018=ORIENTED_EDGE('',*,*,#14585,.T.);
#20019=ORIENTED_EDGE('',*,*,#14526,.F.);
#20020=ORIENTED_EDGE('',*,*,#14586,.T.);
#20021=ORIENTED_EDGE('',*,*,#14488,.T.);
#20022=ORIENTED_EDGE('',*,*,#14587,.T.);
#20023=ORIENTED_EDGE('',*,*,#14496,.T.);
#20024=ORIENTED_EDGE('',*,*,#14588,.T.);
#20025=ORIENTED_EDGE('',*,*,#14518,.F.);
#20026=ORIENTED_EDGE('',*,*,#14589,.T.);
#20027=ORIENTED_EDGE('',*,*,#14525,.F.);
#20028=ORIENTED_EDGE('',*,*,#14554,.F.);
#20029=ORIENTED_EDGE('',*,*,#14489,.F.);
#20030=ORIENTED_EDGE('',*,*,#14586,.F.);
#20031=ORIENTED_EDGE('',*,*,#14491,.F.);
#20032=ORIENTED_EDGE('',*,*,#14555,.F.);
#20033=ORIENTED_EDGE('',*,*,#14523,.F.);
#20034=ORIENTED_EDGE('',*,*,#14578,.F.);
#20035=ORIENTED_EDGE('',*,*,#14493,.F.);
#20036=ORIENTED_EDGE('',*,*,#14579,.F.);
#20037=ORIENTED_EDGE('',*,*,#14521,.F.);
#20038=ORIENTED_EDGE('',*,*,#14552,.F.);
#20039=ORIENTED_EDGE('',*,*,#14495,.F.);
#20040=ORIENTED_EDGE('',*,*,#14553,.F.);
#20041=ORIENTED_EDGE('',*,*,#14519,.F.);
#20042=ORIENTED_EDGE('',*,*,#14588,.F.);
#20043=ORIENTED_EDGE('',*,*,#14501,.F.);
#20044=ORIENTED_EDGE('',*,*,#14580,.F.);
#20045=ORIENTED_EDGE('',*,*,#14513,.F.);
#20046=ORIENTED_EDGE('',*,*,#14583,.F.);
#20047=ORIENTED_EDGE('',*,*,#14499,.F.);
#20048=ORIENTED_EDGE('',*,*,#14550,.F.);
#20049=ORIENTED_EDGE('',*,*,#14515,.F.);
#20050=ORIENTED_EDGE('',*,*,#14581,.F.);
#20051=ORIENTED_EDGE('',*,*,#14517,.F.);
#20052=ORIENTED_EDGE('',*,*,#14551,.F.);
#20053=ORIENTED_EDGE('',*,*,#14497,.F.);
#20054=ORIENTED_EDGE('',*,*,#14589,.F.);
#20055=ORIENTED_EDGE('',*,*,#14487,.F.);
#20056=ORIENTED_EDGE('',*,*,#14556,.F.);
#20057=ORIENTED_EDGE('',*,*,#14527,.F.);
#20058=ORIENTED_EDGE('',*,*,#14587,.F.);
#20059=ORIENTED_EDGE('',*,*,#14503,.F.);
#20060=ORIENTED_EDGE('',*,*,#14582,.F.);
#20061=ORIENTED_EDGE('',*,*,#14511,.F.);
#20062=ORIENTED_EDGE('',*,*,#14584,.F.);
#20063=ORIENTED_EDGE('',*,*,#14434,.F.);
#20064=ORIENTED_EDGE('',*,*,#14411,.T.);
#20065=ORIENTED_EDGE('',*,*,#14461,.T.);
#20066=ORIENTED_EDGE('',*,*,#14508,.T.);
#20067=ORIENTED_EDGE('',*,*,#14590,.T.);
#20068=ORIENTED_EDGE('',*,*,#14319,.T.);
#20069=ORIENTED_EDGE('',*,*,#14316,.T.);
#20070=ORIENTED_EDGE('',*,*,#14421,.F.);
#20071=ORIENTED_EDGE('',*,*,#14507,.F.);
#20072=ORIENTED_EDGE('',*,*,#14438,.T.);
#20073=ORIENTED_EDGE('',*,*,#14320,.T.);
#20074=ORIENTED_EDGE('',*,*,#14590,.F.);
#20075=ORIENTED_EDGE('',*,*,#14506,.F.);
#20076=ORIENTED_EDGE('',*,*,#14407,.T.);
#20077=ORIENTED_EDGE('',*,*,#14416,.F.);
#20078=ORIENTED_EDGE('',*,*,#14393,.T.);
#20079=ORIENTED_EDGE('',*,*,#14402,.F.);
#20080=ORIENTED_EDGE('',*,*,#14379,.T.);
#20081=ORIENTED_EDGE('',*,*,#14388,.F.);
#20082=ORIENTED_EDGE('',*,*,#14365,.T.);
#20083=ORIENTED_EDGE('',*,*,#14374,.F.);
#20084=ORIENTED_EDGE('',*,*,#14351,.T.);
#20085=ORIENTED_EDGE('',*,*,#14360,.F.);
#20086=ORIENTED_EDGE('',*,*,#14337,.T.);
#20087=ORIENTED_EDGE('',*,*,#14346,.F.);
#20088=ORIENTED_EDGE('',*,*,#14323,.T.);
#20089=ORIENTED_EDGE('',*,*,#14332,.F.);
#20090=ORIENTED_EDGE('',*,*,#14309,.T.);
#20091=ORIENTED_EDGE('',*,*,#14318,.F.);
#22958=CYLINDRICAL_SURFACE('',#26271,5.50000000000001);
#22959=CYLINDRICAL_SURFACE('',#26274,3.5);
#22960=CYLINDRICAL_SURFACE('',#26285,5.50000000000001);
#22961=CYLINDRICAL_SURFACE('',#26288,3.5);
#22962=CYLINDRICAL_SURFACE('',#26299,5.50000000000001);
#22963=CYLINDRICAL_SURFACE('',#26302,3.5);
#22964=CYLINDRICAL_SURFACE('',#26313,5.50000000000001);
#22965=CYLINDRICAL_SURFACE('',#26316,3.5);
#22966=CYLINDRICAL_SURFACE('',#26327,5.50000000000001);
#22967=CYLINDRICAL_SURFACE('',#26330,3.5);
#22968=CYLINDRICAL_SURFACE('',#26341,5.50000000000001);
#22969=CYLINDRICAL_SURFACE('',#26344,3.5);
#22970=CYLINDRICAL_SURFACE('',#26355,5.5);
#22971=CYLINDRICAL_SURFACE('',#26358,3.5);
#22972=CYLINDRICAL_SURFACE('',#26369,5.5);
#22973=CYLINDRICAL_SURFACE('',#26372,3.5);
#22974=CYLINDRICAL_SURFACE('',#26469,2.3);
#22975=CYLINDRICAL_SURFACE('',#26470,2.3);
#22976=CYLINDRICAL_SURFACE('',#26471,0.5);
#22977=CYLINDRICAL_SURFACE('',#26472,0.5);
#22978=CYLINDRICAL_SURFACE('',#26473,0.5);
#22979=CYLINDRICAL_SURFACE('',#26474,0.5);
#22980=CYLINDRICAL_SURFACE('',#26475,0.5);
#22981=CYLINDRICAL_SURFACE('',#26476,0.5);
#22982=CYLINDRICAL_SURFACE('',#26477,0.5);
#22983=CYLINDRICAL_SURFACE('',#26478,0.5);
#22984=CYLINDRICAL_SURFACE('',#26479,0.999999999999999);
#22985=CYLINDRICAL_SURFACE('',#26485,2.3);
#22986=CYLINDRICAL_SURFACE('',#26486,2.3);
#22987=CYLINDRICAL_SURFACE('',#26487,0.5);
#22988=CYLINDRICAL_SURFACE('',#26488,0.5);
#22989=CYLINDRICAL_SURFACE('',#26489,0.5);
#22990=CYLINDRICAL_SURFACE('',#26490,0.5);
#22991=CYLINDRICAL_SURFACE('',#26491,0.5);
#22992=CYLINDRICAL_SURFACE('',#26492,0.5);
#22993=CYLINDRICAL_SURFACE('',#26493,0.5);
#22994=CYLINDRICAL_SURFACE('',#26494,0.5);
#22995=CYLINDRICAL_SURFACE('',#26495,0.999999999999999);
#23918=ADVANCED_FACE('',(#2926),#22958,.F.);
#23919=ADVANCED_FACE('',(#2927),#22959,.F.);
#23920=ADVANCED_FACE('',(#2928),#22960,.F.);
#23921=ADVANCED_FACE('',(#2929),#22961,.F.);
#23922=ADVANCED_FACE('',(#2930),#22962,.F.);
#23923=ADVANCED_FACE('',(#2931),#22963,.F.);
#23924=ADVANCED_FACE('',(#2932),#22964,.F.);
#23925=ADVANCED_FACE('',(#2933),#22965,.F.);
#23926=ADVANCED_FACE('',(#2934),#22966,.F.);
#23927=ADVANCED_FACE('',(#2935),#22967,.F.);
#23928=ADVANCED_FACE('',(#2936),#22968,.F.);
#23929=ADVANCED_FACE('',(#2937),#22969,.F.);
#23930=ADVANCED_FACE('',(#2938),#22970,.F.);
#23931=ADVANCED_FACE('',(#2939),#22971,.F.);
#23932=ADVANCED_FACE('',(#2940),#22972,.F.);
#23933=ADVANCED_FACE('',(#2941),#22973,.F.);
#23934=ADVANCED_FACE('',(#2942),#1730,.F.);
#23935=ADVANCED_FACE('',(#2943),#1731,.F.);
#23936=ADVANCED_FACE('',(#2944),#1732,.F.);
#23937=ADVANCED_FACE('',(#2945),#1733,.T.);
#23938=ADVANCED_FACE('',(#2946),#1734,.T.);
#23939=ADVANCED_FACE('',(#2947),#1735,.F.);
#23940=ADVANCED_FACE('',(#2948),#1736,.F.);
#23941=ADVANCED_FACE('',(#2949),#1737,.F.);
#23942=ADVANCED_FACE('',(#2950),#1738,.F.);
#23943=ADVANCED_FACE('',(#2951),#1739,.F.);
#23944=ADVANCED_FACE('',(#2952),#1740,.F.);
#23945=ADVANCED_FACE('',(#2953),#1741,.F.);
#23946=ADVANCED_FACE('',(#2954),#1742,.F.);
#23947=ADVANCED_FACE('',(#2955),#1743,.F.);
#23948=ADVANCED_FACE('',(#2956),#1744,.F.);
#23949=ADVANCED_FACE('',(#2957),#1745,.F.);
#23950=ADVANCED_FACE('',(#2958),#1746,.F.);
#23951=ADVANCED_FACE('',(#2959),#1747,.F.);
#23952=ADVANCED_FACE('',(#2960),#1748,.F.);
#23953=ADVANCED_FACE('',(#2961),#1749,.F.);
#23954=ADVANCED_FACE('',(#2962),#1750,.F.);
#23955=ADVANCED_FACE('',(#2963),#1751,.F.);
#23956=ADVANCED_FACE('',(#2964),#1752,.F.);
#23957=ADVANCED_FACE('',(#2965),#1753,.F.);
#23958=ADVANCED_FACE('',(#2966),#1754,.F.);
#23959=ADVANCED_FACE('',(#2967),#1755,.F.);
#23960=ADVANCED_FACE('',(#2968),#1756,.T.);
#23961=ADVANCED_FACE('',(#2969),#1757,.F.);
#23962=ADVANCED_FACE('',(#2970),#1758,.F.);
#23963=ADVANCED_FACE('',(#2971),#1759,.F.);
#23964=ADVANCED_FACE('',(#2972),#1760,.F.);
#23965=ADVANCED_FACE('',(#2973),#1761,.F.);
#23966=ADVANCED_FACE('',(#2974),#1762,.T.);
#23967=ADVANCED_FACE('',(#2975),#1763,.T.);
#23968=ADVANCED_FACE('',(#2976,#1277,#1278,#1279,#1280,#1281,#1282,#1283,
#1284),#1764,.T.);
#23969=ADVANCED_FACE('',(#2977),#1765,.T.);
#23970=ADVANCED_FACE('',(#2978),#1766,.T.);
#23971=ADVANCED_FACE('',(#2979),#1767,.T.);
#23972=ADVANCED_FACE('',(#2980),#1768,.T.);
#23973=ADVANCED_FACE('',(#2981),#1769,.T.);
#23974=ADVANCED_FACE('',(#2982),#1770,.T.);
#23975=ADVANCED_FACE('',(#2983),#1771,.T.);
#23976=ADVANCED_FACE('',(#2984),#22974,.F.);
#23977=ADVANCED_FACE('',(#2985),#22975,.F.);
#23978=ADVANCED_FACE('',(#2986),#22976,.T.);
#23979=ADVANCED_FACE('',(#2987),#22977,.T.);
#23980=ADVANCED_FACE('',(#2988),#22978,.T.);
#23981=ADVANCED_FACE('',(#2989),#22979,.T.);
#23982=ADVANCED_FACE('',(#2990),#22980,.F.);
#23983=ADVANCED_FACE('',(#2991),#22981,.F.);
#23984=ADVANCED_FACE('',(#2992),#22982,.T.);
#23985=ADVANCED_FACE('',(#2993),#22983,.T.);
#23986=ADVANCED_FACE('',(#2994),#22984,.T.);
#23987=ADVANCED_FACE('',(#2995),#1772,.F.);
#23988=ADVANCED_FACE('',(#2996),#1773,.F.);
#23989=ADVANCED_FACE('',(#2997),#1774,.F.);
#23990=ADVANCED_FACE('',(#2998),#1775,.F.);
#23991=ADVANCED_FACE('',(#2999),#1776,.F.);
#23992=ADVANCED_FACE('',(#3000),#22985,.F.);
#23993=ADVANCED_FACE('',(#3001),#22986,.F.);
#23994=ADVANCED_FACE('',(#3002),#22987,.T.);
#23995=ADVANCED_FACE('',(#3003),#22988,.T.);
#23996=ADVANCED_FACE('',(#3004),#22989,.T.);
#23997=ADVANCED_FACE('',(#3005),#22990,.T.);
#23998=ADVANCED_FACE('',(#3006),#22991,.F.);
#23999=ADVANCED_FACE('',(#3007),#22992,.F.);
#24000=ADVANCED_FACE('',(#3008),#22993,.T.);
#24001=ADVANCED_FACE('',(#3009),#22994,.T.);
#24002=ADVANCED_FACE('',(#3010),#22995,.T.);
#24003=ADVANCED_FACE('',(#3011),#1777,.F.);
#24004=ADVANCED_FACE('',(#3012),#1778,.F.);
#24005=ADVANCED_FACE('',(#3013),#1779,.F.);
#24006=ADVANCED_FACE('',(#3014,#1285),#1780,.F.);
#24007=ADVANCED_FACE('',(#3015,#1286),#1781,.F.);
#24008=ADVANCED_FACE('',(#3016,#1287),#1782,.F.);
#24009=ADVANCED_FACE('',(#3017,#1288),#1783,.F.);
#24010=ADVANCED_FACE('',(#3018,#1289),#1784,.F.);
#24011=ADVANCED_FACE('',(#3019,#1290),#1785,.F.);
#24012=ADVANCED_FACE('',(#3020,#1291),#1786,.F.);
#24013=ADVANCED_FACE('',(#3021,#1292),#1787,.F.);
#24550=CLOSED_SHELL('',(#23918,#23919,#23920,#23921,#23922,#23923,#23924,
#23925,#23926,#23927,#23928,#23929,#23930,#23931,#23932,#23933,#23934,#23935,
#23936,#23937,#23938,#23939,#23940,#23941,#23942,#23943,#23944,#23945,#23946,
#23947,#23948,#23949,#23950,#23951,#23952,#23953,#23954,#23955,#23956,#23957,
#23958,#23959,#23960,#23961,#23962,#23963,#23964,#23965,#23966,#23967,#23968,
#23969,#23970,#23971,#23972,#23973,#23974,#23975,#23976,#23977,#23978,#23979,
#23980,#23981,#23982,#23983,#23984,#23985,#23986,#23987,#23988,#23989,#23990,
#23991,#23992,#23993,#23994,#23995,#23996,#23997,#23998,#23999,#24000,#24001,
#24002,#24003,#24004,#24005,#24006,#24007,#24008,#24009,#24010,#24011,#24012,
#24013));
#26270=AXIS2_PLACEMENT_3D('',#53469,#31163,#31164);
#26271=AXIS2_PLACEMENT_3D('',#53470,#31165,#31166);
#26272=AXIS2_PLACEMENT_3D('',#53472,#31167,#31168);
#26273=AXIS2_PLACEMENT_3D('',#53475,#31170,#31171);
#26274=AXIS2_PLACEMENT_3D('',#53476,#31172,#31173);
#26275=AXIS2_PLACEMENT_3D('',#53479,#31174,#31175);
#26276=AXIS2_PLACEMENT_3D('',#53481,#31176,#31177);
#26277=AXIS2_PLACEMENT_3D('',#53483,#31178,#31179);
#26278=AXIS2_PLACEMENT_3D('',#53485,#31180,#31181);
#26279=AXIS2_PLACEMENT_3D('',#53487,#31182,#31183);
#26280=AXIS2_PLACEMENT_3D('',#53490,#31185,#31186);
#26281=AXIS2_PLACEMENT_3D('',#53492,#31187,#31188);
#26282=AXIS2_PLACEMENT_3D('',#53494,#31189,#31190);
#26283=AXIS2_PLACEMENT_3D('',#53496,#31191,#31192);
#26284=AXIS2_PLACEMENT_3D('',#53497,#31193,#31194);
#26285=AXIS2_PLACEMENT_3D('',#53498,#31195,#31196);
#26286=AXIS2_PLACEMENT_3D('',#53500,#31197,#31198);
#26287=AXIS2_PLACEMENT_3D('',#53503,#31200,#31201);
#26288=AXIS2_PLACEMENT_3D('',#53504,#31202,#31203);
#26289=AXIS2_PLACEMENT_3D('',#53507,#31204,#31205);
#26290=AXIS2_PLACEMENT_3D('',#53509,#31206,#31207);
#26291=AXIS2_PLACEMENT_3D('',#53511,#31208,#31209);
#26292=AXIS2_PLACEMENT_3D('',#53513,#31210,#31211);
#26293=AXIS2_PLACEMENT_3D('',#53515,#31212,#31213);
#26294=AXIS2_PLACEMENT_3D('',#53518,#31215,#31216);
#26295=AXIS2_PLACEMENT_3D('',#53520,#31217,#31218);
#26296=AXIS2_PLACEMENT_3D('',#53522,#31219,#31220);
#26297=AXIS2_PLACEMENT_3D('',#53524,#31221,#31222);
#26298=AXIS2_PLACEMENT_3D('',#53525,#31223,#31224);
#26299=AXIS2_PLACEMENT_3D('',#53526,#31225,#31226);
#26300=AXIS2_PLACEMENT_3D('',#53528,#31227,#31228);
#26301=AXIS2_PLACEMENT_3D('',#53531,#31230,#31231);
#26302=AXIS2_PLACEMENT_3D('',#53532,#31232,#31233);
#26303=AXIS2_PLACEMENT_3D('',#53535,#31234,#31235);
#26304=AXIS2_PLACEMENT_3D('',#53537,#31236,#31237);
#26305=AXIS2_PLACEMENT_3D('',#53539,#31238,#31239);
#26306=AXIS2_PLACEMENT_3D('',#53541,#31240,#31241);
#26307=AXIS2_PLACEMENT_3D('',#53543,#31242,#31243);
#26308=AXIS2_PLACEMENT_3D('',#53546,#31245,#31246);
#26309=AXIS2_PLACEMENT_3D('',#53548,#31247,#31248);
#26310=AXIS2_PLACEMENT_3D('',#53550,#31249,#31250);
#26311=AXIS2_PLACEMENT_3D('',#53552,#31251,#31252);
#26312=AXIS2_PLACEMENT_3D('',#53553,#31253,#31254);
#26313=AXIS2_PLACEMENT_3D('',#53554,#31255,#31256);
#26314=AXIS2_PLACEMENT_3D('',#53556,#31257,#31258);
#26315=AXIS2_PLACEMENT_3D('',#53559,#31260,#31261);
#26316=AXIS2_PLACEMENT_3D('',#53560,#31262,#31263);
#26317=AXIS2_PLACEMENT_3D('',#53563,#31264,#31265);
#26318=AXIS2_PLACEMENT_3D('',#53565,#31266,#31267);
#26319=AXIS2_PLACEMENT_3D('',#53567,#31268,#31269);
#26320=AXIS2_PLACEMENT_3D('',#53569,#31270,#31271);
#26321=AXIS2_PLACEMENT_3D('',#53571,#31272,#31273);
#26322=AXIS2_PLACEMENT_3D('',#53574,#31275,#31276);
#26323=AXIS2_PLACEMENT_3D('',#53576,#31277,#31278);
#26324=AXIS2_PLACEMENT_3D('',#53578,#31279,#31280);
#26325=AXIS2_PLACEMENT_3D('',#53580,#31281,#31282);
#26326=AXIS2_PLACEMENT_3D('',#53581,#31283,#31284);
#26327=AXIS2_PLACEMENT_3D('',#53582,#31285,#31286);
#26328=AXIS2_PLACEMENT_3D('',#53584,#31287,#31288);
#26329=AXIS2_PLACEMENT_3D('',#53587,#31290,#31291);
#26330=AXIS2_PLACEMENT_3D('',#53588,#31292,#31293);
#26331=AXIS2_PLACEMENT_3D('',#53591,#31294,#31295);
#26332=AXIS2_PLACEMENT_3D('',#53593,#31296,#31297);
#26333=AXIS2_PLACEMENT_3D('',#53595,#31298,#31299);
#26334=AXIS2_PLACEMENT_3D('',#53597,#31300,#31301);
#26335=AXIS2_PLACEMENT_3D('',#53599,#31302,#31303);
#26336=AXIS2_PLACEMENT_3D('',#53602,#31305,#31306);
#26337=AXIS2_PLACEMENT_3D('',#53604,#31307,#31308);
#26338=AXIS2_PLACEMENT_3D('',#53606,#31309,#31310);
#26339=AXIS2_PLACEMENT_3D('',#53608,#31311,#31312);
#26340=AXIS2_PLACEMENT_3D('',#53609,#31313,#31314);
#26341=AXIS2_PLACEMENT_3D('',#53610,#31315,#31316);
#26342=AXIS2_PLACEMENT_3D('',#53612,#31317,#31318);
#26343=AXIS2_PLACEMENT_3D('',#53615,#31320,#31321);
#26344=AXIS2_PLACEMENT_3D('',#53616,#31322,#31323);
#26345=AXIS2_PLACEMENT_3D('',#53619,#31324,#31325);
#26346=AXIS2_PLACEMENT_3D('',#53621,#31326,#31327);
#26347=AXIS2_PLACEMENT_3D('',#53623,#31328,#31329);
#26348=AXIS2_PLACEMENT_3D('',#53625,#31330,#31331);
#26349=AXIS2_PLACEMENT_3D('',#53627,#31332,#31333);
#26350=AXIS2_PLACEMENT_3D('',#53630,#31335,#31336);
#26351=AXIS2_PLACEMENT_3D('',#53632,#31337,#31338);
#26352=AXIS2_PLACEMENT_3D('',#53634,#31339,#31340);
#26353=AXIS2_PLACEMENT_3D('',#53636,#31341,#31342);
#26354=AXIS2_PLACEMENT_3D('',#53637,#31343,#31344);
#26355=AXIS2_PLACEMENT_3D('',#53638,#31345,#31346);
#26356=AXIS2_PLACEMENT_3D('',#53640,#31347,#31348);
#26357=AXIS2_PLACEMENT_3D('',#53643,#31350,#31351);
#26358=AXIS2_PLACEMENT_3D('',#53644,#31352,#31353);
#26359=AXIS2_PLACEMENT_3D('',#53647,#31354,#31355);
#26360=AXIS2_PLACEMENT_3D('',#53649,#31356,#31357);
#26361=AXIS2_PLACEMENT_3D('',#53651,#31358,#31359);
#26362=AXIS2_PLACEMENT_3D('',#53653,#31360,#31361);
#26363=AXIS2_PLACEMENT_3D('',#53655,#31362,#31363);
#26364=AXIS2_PLACEMENT_3D('',#53658,#31365,#31366);
#26365=AXIS2_PLACEMENT_3D('',#53660,#31367,#31368);
#26366=AXIS2_PLACEMENT_3D('',#53662,#31369,#31370);
#26367=AXIS2_PLACEMENT_3D('',#53664,#31371,#31372);
#26368=AXIS2_PLACEMENT_3D('',#53665,#31373,#31374);
#26369=AXIS2_PLACEMENT_3D('',#53666,#31375,#31376);
#26370=AXIS2_PLACEMENT_3D('',#53668,#31377,#31378);
#26371=AXIS2_PLACEMENT_3D('',#53671,#31380,#31381);
#26372=AXIS2_PLACEMENT_3D('',#53672,#31382,#31383);
#26373=AXIS2_PLACEMENT_3D('',#53675,#31384,#31385);
#26374=AXIS2_PLACEMENT_3D('',#53677,#31386,#31387);
#26375=AXIS2_PLACEMENT_3D('',#53679,#31388,#31389);
#26376=AXIS2_PLACEMENT_3D('',#53681,#31390,#31391);
#26377=AXIS2_PLACEMENT_3D('',#53683,#31392,#31393);
#26378=AXIS2_PLACEMENT_3D('',#53686,#31395,#31396);
#26379=AXIS2_PLACEMENT_3D('',#53688,#31397,#31398);
#26380=AXIS2_PLACEMENT_3D('',#53690,#31399,#31400);
#26381=AXIS2_PLACEMENT_3D('',#53692,#31401,#31402);
#26382=AXIS2_PLACEMENT_3D('',#53693,#31403,#31404);
#26383=AXIS2_PLACEMENT_3D('',#53694,#31405,#31406);
#26384=AXIS2_PLACEMENT_3D('',#53700,#31410,#31411);
#26385=AXIS2_PLACEMENT_3D('',#53703,#31414,#31415);
#26386=AXIS2_PLACEMENT_3D('',#53705,#31417,#31418);
#26387=AXIS2_PLACEMENT_3D('',#53720,#31430,#31431);
#26388=AXIS2_PLACEMENT_3D('',#53736,#31443,#31444);
#26389=AXIS2_PLACEMENT_3D('',#53737,#31445,#31446);
#26390=AXIS2_PLACEMENT_3D('',#53740,#31449,#31450);
#26391=AXIS2_PLACEMENT_3D('',#53741,#31451,#31452);
#26392=AXIS2_PLACEMENT_3D('',#53742,#31453,#31454);
#26393=AXIS2_PLACEMENT_3D('',#53745,#31457,#31458);
#26394=AXIS2_PLACEMENT_3D('',#53746,#31459,#31460);
#26395=AXIS2_PLACEMENT_3D('',#53747,#31461,#31462);
#26396=AXIS2_PLACEMENT_3D('',#53749,#31464,#31465);
#26397=AXIS2_PLACEMENT_3D('',#53751,#31467,#31468);
#26398=AXIS2_PLACEMENT_3D('',#53752,#31469,#31470);
#26399=AXIS2_PLACEMENT_3D('',#53755,#31473,#31474);
#26400=AXIS2_PLACEMENT_3D('',#53756,#31475,#31476);
#26401=AXIS2_PLACEMENT_3D('',#53757,#31477,#31478);
#26402=AXIS2_PLACEMENT_3D('',#53760,#31481,#31482);
#26403=AXIS2_PLACEMENT_3D('',#53761,#31483,#31484);
#26404=AXIS2_PLACEMENT_3D('',#53762,#31485,#31486);
#26405=AXIS2_PLACEMENT_3D('',#53765,#31489,#31490);
#26406=AXIS2_PLACEMENT_3D('',#53766,#31491,#31492);
#26407=AXIS2_PLACEMENT_3D('',#53767,#31493,#31494);
#26408=AXIS2_PLACEMENT_3D('',#53773,#31498,#31499);
#26409=AXIS2_PLACEMENT_3D('',#53775,#31501,#31502);
#26410=AXIS2_PLACEMENT_3D('',#53781,#31505,#31506);
#26411=AXIS2_PLACEMENT_3D('',#53785,#31508,#31509);
#26412=AXIS2_PLACEMENT_3D('',#53789,#31511,#31512);
#26413=AXIS2_PLACEMENT_3D('',#53793,#31514,#31515);
#26414=AXIS2_PLACEMENT_3D('',#53795,#31516,#31517);
#26415=AXIS2_PLACEMENT_3D('',#53797,#31518,#31519);
#26416=AXIS2_PLACEMENT_3D('',#53801,#31521,#31522);
#26417=AXIS2_PLACEMENT_3D('',#53805,#31524,#31525);
#26418=AXIS2_PLACEMENT_3D('',#53809,#31527,#31528);
#26419=AXIS2_PLACEMENT_3D('',#53811,#31529,#31530);
#26420=AXIS2_PLACEMENT_3D('',#53813,#31531,#31532);
#26421=AXIS2_PLACEMENT_3D('',#53821,#31536,#31537);
#26422=AXIS2_PLACEMENT_3D('',#53823,#31538,#31539);
#26423=AXIS2_PLACEMENT_3D('',#53825,#31540,#31541);
#26424=AXIS2_PLACEMENT_3D('',#53829,#31543,#31544);
#26425=AXIS2_PLACEMENT_3D('',#53833,#31546,#31547);
#26426=AXIS2_PLACEMENT_3D('',#53837,#31549,#31550);
#26427=AXIS2_PLACEMENT_3D('',#53839,#31551,#31552);
#26428=AXIS2_PLACEMENT_3D('',#53841,#31553,#31554);
#26429=AXIS2_PLACEMENT_3D('',#53845,#31556,#31557);
#26430=AXIS2_PLACEMENT_3D('',#53849,#31559,#31560);
#26431=AXIS2_PLACEMENT_3D('',#53853,#31562,#31563);
#26432=AXIS2_PLACEMENT_3D('',#53860,#31568,#31569);
#26433=AXIS2_PLACEMENT_3D('',#53867,#31573,#31574);
#26434=AXIS2_PLACEMENT_3D('',#53871,#31576,#31577);
#26435=AXIS2_PLACEMENT_3D('',#53875,#31579,#31580);
#26436=AXIS2_PLACEMENT_3D('',#53879,#31582,#31583);
#26437=AXIS2_PLACEMENT_3D('',#53881,#31584,#31585);
#26438=AXIS2_PLACEMENT_3D('',#53883,#31586,#31587);
#26439=AXIS2_PLACEMENT_3D('',#53887,#31589,#31590);
#26440=AXIS2_PLACEMENT_3D('',#53891,#31592,#31593);
#26441=AXIS2_PLACEMENT_3D('',#53895,#31595,#31596);
#26442=AXIS2_PLACEMENT_3D('',#53897,#31597,#31598);
#26443=AXIS2_PLACEMENT_3D('',#53899,#31599,#31600);
#26444=AXIS2_PLACEMENT_3D('',#53907,#31604,#31605);
#26445=AXIS2_PLACEMENT_3D('',#53909,#31606,#31607);
#26446=AXIS2_PLACEMENT_3D('',#53911,#31608,#31609);
#26447=AXIS2_PLACEMENT_3D('',#53915,#31611,#31612);
#26448=AXIS2_PLACEMENT_3D('',#53919,#31614,#31615);
#26449=AXIS2_PLACEMENT_3D('',#53923,#31617,#31618);
#26450=AXIS2_PLACEMENT_3D('',#53925,#31619,#31620);
#26451=AXIS2_PLACEMENT_3D('',#53927,#31621,#31622);
#26452=AXIS2_PLACEMENT_3D('',#53931,#31624,#31625);
#26453=AXIS2_PLACEMENT_3D('',#53935,#31627,#31628);
#26454=AXIS2_PLACEMENT_3D('',#53939,#31630,#31631);
#26455=AXIS2_PLACEMENT_3D('',#53943,#31634,#31635);
#26456=AXIS2_PLACEMENT_3D('',#53946,#31638,#31639);
#26457=AXIS2_PLACEMENT_3D('',#53949,#31642,#31643);
#26458=AXIS2_PLACEMENT_3D('',#53952,#31646,#31647);
#26459=AXIS2_PLACEMENT_3D('',#53955,#31650,#31651);
#26460=AXIS2_PLACEMENT_3D('',#53958,#31654,#31655);
#26461=AXIS2_PLACEMENT_3D('',#53961,#31658,#31659);
#26462=AXIS2_PLACEMENT_3D('',#53963,#31661,#31662);
#26463=AXIS2_PLACEMENT_3D('',#53965,#31664,#31665);
#26464=AXIS2_PLACEMENT_3D('',#53967,#31667,#31668);
#26465=AXIS2_PLACEMENT_3D('',#53970,#31671,#31672);
#26466=AXIS2_PLACEMENT_3D('',#53973,#31675,#31676);
#26467=AXIS2_PLACEMENT_3D('',#53976,#31679,#31680);
#26468=AXIS2_PLACEMENT_3D('',#53979,#31683,#31684);
#26469=AXIS2_PLACEMENT_3D('',#53981,#31686,#31687);
#26470=AXIS2_PLACEMENT_3D('',#53984,#31690,#31691);
#26471=AXIS2_PLACEMENT_3D('',#53987,#31694,#31695);
#26472=AXIS2_PLACEMENT_3D('',#53988,#31696,#31697);
#26473=AXIS2_PLACEMENT_3D('',#53989,#31698,#31699);
#26474=AXIS2_PLACEMENT_3D('',#53990,#31700,#31701);
#26475=AXIS2_PLACEMENT_3D('',#53991,#31702,#31703);
#26476=AXIS2_PLACEMENT_3D('',#53992,#31704,#31705);
#26477=AXIS2_PLACEMENT_3D('',#53993,#31706,#31707);
#26478=AXIS2_PLACEMENT_3D('',#53994,#31708,#31709);
#26479=AXIS2_PLACEMENT_3D('',#53995,#31710,#31711);
#26480=AXIS2_PLACEMENT_3D('',#53996,#31712,#31713);
#26481=AXIS2_PLACEMENT_3D('',#53999,#31716,#31717);
#26482=AXIS2_PLACEMENT_3D('',#54002,#31720,#31721);
#26483=AXIS2_PLACEMENT_3D('',#54005,#31724,#31725);
#26484=AXIS2_PLACEMENT_3D('',#54008,#31728,#31729);
#26485=AXIS2_PLACEMENT_3D('',#54009,#31730,#31731);
#26486=AXIS2_PLACEMENT_3D('',#54012,#31734,#31735);
#26487=AXIS2_PLACEMENT_3D('',#54015,#31738,#31739);
#26488=AXIS2_PLACEMENT_3D('',#54016,#31740,#31741);
#26489=AXIS2_PLACEMENT_3D('',#54017,#31742,#31743);
#26490=AXIS2_PLACEMENT_3D('',#54018,#31744,#31745);
#26491=AXIS2_PLACEMENT_3D('',#54019,#31746,#31747);
#26492=AXIS2_PLACEMENT_3D('',#54020,#31748,#31749);
#26493=AXIS2_PLACEMENT_3D('',#54021,#31750,#31751);
#26494=AXIS2_PLACEMENT_3D('',#54022,#31752,#31753);
#26495=AXIS2_PLACEMENT_3D('',#54023,#31754,#31755);
#26496=AXIS2_PLACEMENT_3D('',#54024,#31756,#31757);
#26497=AXIS2_PLACEMENT_3D('',#54025,#31758,#31759);
#26498=AXIS2_PLACEMENT_3D('',#54027,#31761,#31762);
#26499=AXIS2_PLACEMENT_3D('',#54028,#31763,#31764);
#26500=AXIS2_PLACEMENT_3D('',#54029,#31765,#31766);
#26501=AXIS2_PLACEMENT_3D('',#54030,#31767,#31768);
#26502=AXIS2_PLACEMENT_3D('',#54031,#31769,#31770);
#26503=AXIS2_PLACEMENT_3D('',#54032,#31771,#31772);
#26504=AXIS2_PLACEMENT_3D('',#54033,#31773,#31774);
#26505=AXIS2_PLACEMENT_3D('',#54034,#31775,#31776);
#26506=AXIS2_PLACEMENT_3D('',#54035,#31777,#31778);
#31163=DIRECTION('axis',(0.,0.,1.));
#31164=DIRECTION('refdir',(1.,0.,0.));
#31165=DIRECTION('center_axis',(0.,1.,0.));
#31166=DIRECTION('ref_axis',(0.,0.,1.));
#31167=DIRECTION('center_axis',(0.,1.,0.));
#31168=DIRECTION('ref_axis',(0.,0.,1.));
#31169=DIRECTION('',(0.,1.,0.));
#31170=DIRECTION('center_axis',(0.,1.,0.));
#31171=DIRECTION('ref_axis',(0.,0.,1.));
#31172=DIRECTION('center_axis',(0.,1.,0.));
#31173=DIRECTION('ref_axis',(0.,0.,1.));
#31174=DIRECTION('center_axis',(6.19544098563146E-17,1.,0.));
#31175=DIRECTION('ref_axis',(-1.,6.19544098563145E-17,0.));
#31176=DIRECTION('center_axis',(-0.707106781186515,0.70710678118658,-8.91973620485813E-14));
#31177=DIRECTION('ref_axis',(0.70710678118658,0.707106781186515,-4.06869792218931E-9));
#31178=DIRECTION('center_axis',(0.,1.,0.));
#31179=DIRECTION('ref_axis',(0.,0.,1.));
#31180=DIRECTION('center_axis',(-0.707106781186512,0.707106781186583,1.02279641815266E-13));
#31181=DIRECTION('ref_axis',(0.707106781186583,0.707106781186512,-1.02741687219779E-8));
#31182=DIRECTION('center_axis',(6.19544098563146E-17,1.,0.));
#31183=DIRECTION('ref_axis',(-1.,6.19544098563145E-17,0.));
#31184=DIRECTION('',(0.,1.,0.));
#31185=DIRECTION('center_axis',(0.,1.,0.));
#31186=DIRECTION('ref_axis',(0.,0.,1.));
#31187=DIRECTION('center_axis',(6.19544098563146E-17,1.,0.));
#31188=DIRECTION('ref_axis',(-1.,6.19544098563145E-17,0.));
#31189=DIRECTION('center_axis',(0.707106781186576,0.707106781186519,-7.49257841204838E-14));
#31190=DIRECTION('ref_axis',(0.707106781186519,-0.707106781186576,-8.08586735251008E-9));
#31191=DIRECTION('center_axis',(0.,1.,0.));
#31192=DIRECTION('ref_axis',(0.,0.,1.));
#31193=DIRECTION('center_axis',(0.707106781186584,0.707106781186511,9.99010454948653E-14));
#31194=DIRECTION('ref_axis',(0.707106781186511,-0.707106781186585,-3.84531478187653E-9));
#31195=DIRECTION('center_axis',(0.,1.,0.));
#31196=DIRECTION('ref_axis',(0.,0.,1.));
#31197=DIRECTION('center_axis',(0.,1.,0.));
#31198=DIRECTION('ref_axis',(0.,0.,1.));
#31199=DIRECTION('',(0.,1.,0.));
#31200=DIRECTION('center_axis',(0.,1.,0.));
#31201=DIRECTION('ref_axis',(0.,0.,1.));
#31202=DIRECTION('center_axis',(0.,1.,0.));
#31203=DIRECTION('ref_axis',(0.,0.,1.));
#31204=DIRECTION('center_axis',(6.19544098563146E-17,1.,0.));
#31205=DIRECTION('ref_axis',(-1.,6.19544098563145E-17,0.));
#31206=DIRECTION('center_axis',(-0.707106781186517,0.707106781186578,-8.56294675662794E-14));
#31207=DIRECTION('ref_axis',(0.707106781186578,0.707106781186517,6.04191337821136E-9));
#31208=DIRECTION('center_axis',(0.,1.,0.));
#31209=DIRECTION('ref_axis',(0.,0.,1.));
#31210=DIRECTION('center_axis',(-0.707106781186516,0.707106781186579,8.80080638879547E-14));
#31211=DIRECTION('ref_axis',(0.707106781186579,0.707106781186516,-1.3593282001024E-10));
#31212=DIRECTION('center_axis',(6.19544098563146E-17,1.,0.));
#31213=DIRECTION('ref_axis',(-1.,6.19544098563145E-17,0.));
#31214=DIRECTION('',(0.,1.,0.));
#31215=DIRECTION('center_axis',(0.,1.,0.));
#31216=DIRECTION('ref_axis',(0.,0.,1.));
#31217=DIRECTION('center_axis',(6.19544098563146E-17,1.,0.));
#31218=DIRECTION('ref_axis',(-1.,6.19544098563145E-17,0.));
#31219=DIRECTION('center_axis',(0.707106781186558,0.707106781186537,-1.42715779277089E-14));
#31220=DIRECTION('ref_axis',(0.707106781186537,-0.707106781186558,-6.58917923406118E-10));
#31221=DIRECTION('center_axis',(0.,1.,0.));
#31222=DIRECTION('ref_axis',(0.,0.,1.));
#31223=DIRECTION('center_axis',(0.70710678118656,0.707106781186535,2.37859632128526E-14));
#31224=DIRECTION('ref_axis',(0.707106781186535,-0.70710678118656,1.32329140713553E-8));
#31225=DIRECTION('center_axis',(0.,1.,0.));
#31226=DIRECTION('ref_axis',(0.,0.,1.));
#31227=DIRECTION('center_axis',(0.,1.,0.));
#31228=DIRECTION('ref_axis',(0.,0.,1.));
#31229=DIRECTION('',(0.,1.,0.));
#31230=DIRECTION('center_axis',(0.,1.,0.));
#31231=DIRECTION('ref_axis',(0.,0.,1.));
#31232=DIRECTION('center_axis',(0.,1.,0.));
#31233=DIRECTION('ref_axis',(0.,0.,1.));
#31234=DIRECTION('center_axis',(6.19544098563146E-17,1.,0.));
#31235=DIRECTION('ref_axis',(-1.,6.19544098563145E-17,0.));
#31236=DIRECTION('center_axis',(-0.707106781186517,0.707106781186578,-8.56294675664632E-14));
#31237=DIRECTION('ref_axis',(0.707106781186578,0.707106781186517,2.05409793046914E-10));
#31238=DIRECTION('center_axis',(0.,1.,0.));
#31239=DIRECTION('ref_axis',(0.,0.,1.));
#31240=DIRECTION('center_axis',(-0.707106781186514,0.707106781186581,9.51438528521397E-14));
#31241=DIRECTION('ref_axis',(0.707106781186581,0.707106781186514,-1.68463230688698E-9));
#31242=DIRECTION('center_axis',(6.19544098563146E-17,1.,0.));
#31243=DIRECTION('ref_axis',(-1.,6.19544098563145E-17,0.));
#31244=DIRECTION('',(0.,1.,0.));
#31245=DIRECTION('center_axis',(0.,1.,0.));
#31246=DIRECTION('ref_axis',(0.,0.,1.));
#31247=DIRECTION('center_axis',(6.19544098563146E-17,1.,0.));
#31248=DIRECTION('ref_axis',(-1.,6.19544098563145E-17,0.));
#31249=DIRECTION('center_axis',(0.707106781186562,0.707106781186533,-2.7353857695029E-14));
#31250=DIRECTION('ref_axis',(0.707106781186533,-0.707106781186562,3.81701637658264E-9));
#31251=DIRECTION('center_axis',(0.,1.,0.));
#31252=DIRECTION('ref_axis',(0.,0.,1.));
#31253=DIRECTION('center_axis',(0.707106781186559,0.707106781186536,1.90287705704185E-14));
#31254=DIRECTION('ref_axis',(0.707106781186536,-0.707106781186559,-1.36144986195536E-8));
#31255=DIRECTION('center_axis',(0.,1.,0.));
#31256=DIRECTION('ref_axis',(0.,0.,1.));
#31257=DIRECTION('center_axis',(0.,1.,0.));
#31258=DIRECTION('ref_axis',(0.,0.,1.));
#31259=DIRECTION('',(0.,1.,0.));
#31260=DIRECTION('center_axis',(0.,1.,0.));
#31261=DIRECTION('ref_axis',(0.,0.,1.));
#31262=DIRECTION('center_axis',(0.,1.,0.));
#31263=DIRECTION('ref_axis',(0.,0.,1.));
#31264=DIRECTION('center_axis',(6.19544098563146E-17,1.,0.));
#31265=DIRECTION('ref_axis',(-1.,6.19544098563145E-17,0.));
#31266=DIRECTION('center_axis',(-0.707106781186512,0.707106781186583,-1.01090343655035E-13));
#31267=DIRECTION('ref_axis',(0.707106781186583,0.707106781186512,-6.95106205771872E-9));
#31268=DIRECTION('center_axis',(0.,1.,0.));
#31269=DIRECTION('ref_axis',(0.,0.,1.));
#31270=DIRECTION('center_axis',(-0.707106781186507,0.707106781186588,1.11794027100389E-13));
#31271=DIRECTION('ref_axis',(0.707106781186588,0.707106781186507,-1.20597831914651E-9));
#31272=DIRECTION('center_axis',(6.19544098563146E-17,1.,0.));
#31273=DIRECTION('ref_axis',(-1.,6.19544098563145E-17,0.));
#31274=DIRECTION('',(0.,1.,0.));
#31275=DIRECTION('center_axis',(0.,1.,0.));
#31276=DIRECTION('ref_axis',(0.,0.,1.));
#31277=DIRECTION('center_axis',(6.19544098563146E-17,1.,0.));
#31278=DIRECTION('ref_axis',(-1.,6.19544098563145E-17,0.));
#31279=DIRECTION('center_axis',(0.707106781186587,0.707106781186508,-1.03468939976327E-13));
#31280=DIRECTION('ref_axis',(0.707106781186508,-0.707106781186587,-1.2458919406139E-9));
#31281=DIRECTION('center_axis',(0.,1.,0.));
#31282=DIRECTION('ref_axis',(0.,0.,1.));
#31283=DIRECTION('center_axis',(0.707106781186591,0.707106781186504,1.21308412386573E-13));
#31284=DIRECTION('ref_axis',(0.707106781186504,-0.707106781186591,-3.13413565581154E-9));
#31285=DIRECTION('center_axis',(0.,1.,0.));
#31286=DIRECTION('ref_axis',(0.,0.,1.));
#31287=DIRECTION('center_axis',(0.,1.,0.));
#31288=DIRECTION('ref_axis',(0.,0.,1.));
#31289=DIRECTION('',(0.,1.,0.));
#31290=DIRECTION('center_axis',(0.,1.,0.));
#31291=DIRECTION('ref_axis',(0.,0.,1.));
#31292=DIRECTION('center_axis',(0.,1.,0.));
#31293=DIRECTION('ref_axis',(0.,0.,1.));
#31294=DIRECTION('center_axis',(6.19544098563146E-17,1.,0.));
#31295=DIRECTION('ref_axis',(-1.,6.19544098563145E-17,0.));
#31296=DIRECTION('center_axis',(-0.707106781186512,0.707106781186583,-1.01090343655035E-13));
#31297=DIRECTION('ref_axis',(0.707106781186583,0.707106781186512,-4.84274768749914E-9));
#31298=DIRECTION('center_axis',(0.,1.,0.));
#31299=DIRECTION('ref_axis',(0.,0.,1.));
#31300=DIRECTION('center_axis',(-0.707106781186507,0.707106781186588,1.11794027100512E-13));
#31301=DIRECTION('ref_axis',(0.707106781186588,0.707106781186507,-5.79440054969364E-10));
#31302=DIRECTION('center_axis',(6.19544098563146E-17,1.,0.));
#31303=DIRECTION('ref_axis',(-1.,6.19544098563145E-17,0.));
#31304=DIRECTION('',(0.,1.,0.));
#31305=DIRECTION('center_axis',(0.,1.,0.));
#31306=DIRECTION('ref_axis',(0.,0.,1.));
#31307=DIRECTION('center_axis',(6.19544098563146E-17,1.,0.));
#31308=DIRECTION('ref_axis',(-1.,6.19544098563145E-17,0.));
#31309=DIRECTION('center_axis',(0.707106781186572,0.707106781186523,-6.06542061931958E-14));
#31310=DIRECTION('ref_axis',(0.707106781186523,-0.707106781186572,-4.16681478047922E-10));
#31311=DIRECTION('center_axis',(0.,1.,0.));
#31312=DIRECTION('ref_axis',(0.,0.,1.));
#31313=DIRECTION('center_axis',(0.707106781186573,0.707106781186523,5.94649080322994E-14));
#31314=DIRECTION('ref_axis',(0.707106781186522,-0.707106781186572,-7.07966748929713E-9));
#31315=DIRECTION('center_axis',(0.,1.,0.));
#31316=DIRECTION('ref_axis',(0.,0.,1.));
#31317=DIRECTION('center_axis',(0.,1.,0.));
#31318=DIRECTION('ref_axis',(0.,0.,1.));
#31319=DIRECTION('',(0.,1.,0.));
#31320=DIRECTION('center_axis',(0.,1.,0.));
#31321=DIRECTION('ref_axis',(0.,0.,1.));
#31322=DIRECTION('center_axis',(0.,1.,0.));
#31323=DIRECTION('ref_axis',(0.,0.,1.));
#31324=DIRECTION('center_axis',(6.19544098563146E-17,1.,0.));
#31325=DIRECTION('ref_axis',(-1.,6.19544098563145E-17,0.));
#31326=DIRECTION('center_axis',(-0.707106781186512,0.707106781186583,-9.75224491731711E-14));
#31327=DIRECTION('ref_axis',(0.707106781186583,0.707106781186512,8.28098005345847E-10));
#31328=DIRECTION('center_axis',(0.,1.,0.));
#31329=DIRECTION('ref_axis',(0.,0.,1.));
#31330=DIRECTION('center_axis',(-0.707106781186517,0.707106781186578,8.80080638877943E-14));
#31331=DIRECTION('ref_axis',(0.707106781186578,0.707106781186517,2.21337779031319E-9));
#31332=DIRECTION('center_axis',(6.19544098563146E-17,1.,0.));
#31333=DIRECTION('ref_axis',(-1.,6.19544098563145E-17,0.));
#31334=DIRECTION('',(0.,1.,0.));
#31335=DIRECTION('center_axis',(0.,1.,0.));
#31336=DIRECTION('ref_axis',(0.,0.,1.));
#31337=DIRECTION('center_axis',(6.19544098563146E-17,1.,0.));
#31338=DIRECTION('ref_axis',(-1.,6.19544098563145E-17,0.));
#31339=DIRECTION('center_axis',(0.707106781186559,0.707106781186536,-1.54608760884523E-14));
#31340=DIRECTION('ref_axis',(0.707106781186536,-0.707106781186559,-3.73251907398984E-10));
#31341=DIRECTION('center_axis',(0.,1.,0.));
#31342=DIRECTION('ref_axis',(0.,0.,1.));
#31343=DIRECTION('center_axis',(0.707106781186559,0.707106781186536,2.14073668916763E-14));
#31344=DIRECTION('ref_axis',(0.707106781186536,-0.707106781186559,-2.78541967759128E-9));
#31345=DIRECTION('center_axis',(0.,1.,0.));
#31346=DIRECTION('ref_axis',(0.,0.,1.));
#31347=DIRECTION('center_axis',(0.,1.,0.));
#31348=DIRECTION('ref_axis',(0.,0.,1.));
#31349=DIRECTION('',(0.,1.,0.));
#31350=DIRECTION('center_axis',(0.,1.,0.));
#31351=DIRECTION('ref_axis',(0.,0.,1.));
#31352=DIRECTION('center_axis',(0.,1.,0.));
#31353=DIRECTION('ref_axis',(0.,0.,1.));
#31354=DIRECTION('center_axis',(6.19544098563146E-17,1.,0.));
#31355=DIRECTION('ref_axis',(-1.,6.19544098563145E-17,0.));
#31356=DIRECTION('center_axis',(-0.707106781186531,0.707106781186564,-3.68682429800858E-14));
#31357=DIRECTION('ref_axis',(0.707106781186564,0.707106781186531,1.74894276284856E-9));
#31358=DIRECTION('center_axis',(0.,1.,0.));
#31359=DIRECTION('ref_axis',(0.,0.,1.));
#31360=DIRECTION('center_axis',(-0.707106781186539,0.707106781186556,1.90287705703503E-14));
#31361=DIRECTION('ref_axis',(0.707106781186556,0.707106781186538,1.53190884165236E-9));
#31362=DIRECTION('center_axis',(6.19544098563146E-17,1.,0.));
#31363=DIRECTION('ref_axis',(-1.,6.19544098563145E-17,0.));
#31364=DIRECTION('',(0.,1.,0.));
#31365=DIRECTION('center_axis',(0.,1.,0.));
#31366=DIRECTION('ref_axis',(0.,0.,1.));
#31367=DIRECTION('center_axis',(6.19544098563146E-17,1.,0.));
#31368=DIRECTION('ref_axis',(-1.,6.19544098563145E-17,0.));
#31369=DIRECTION('center_axis',(0.707106781186565,0.70710678118653,-3.68682429801788E-14));
#31370=DIRECTION('ref_axis',(0.70710678118653,-0.707106781186565,-1.95898017545691E-10));
#31371=DIRECTION('center_axis',(0.,1.,0.));
#31372=DIRECTION('ref_axis',(0.,0.,1.));
#31373=DIRECTION('center_axis',(0.707106781186568,0.707106781186527,4.28147337832366E-14));
#31374=DIRECTION('ref_axis',(0.707106781186527,-0.707106781186568,-6.13326237593097E-11));
#31375=DIRECTION('center_axis',(0.,1.,0.));
#31376=DIRECTION('ref_axis',(0.,0.,1.));
#31377=DIRECTION('center_axis',(0.,1.,0.));
#31378=DIRECTION('ref_axis',(0.,0.,1.));
#31379=DIRECTION('',(0.,1.,0.));
#31380=DIRECTION('center_axis',(0.,1.,0.));
#31381=DIRECTION('ref_axis',(0.,0.,1.));
#31382=DIRECTION('center_axis',(0.,1.,0.));
#31383=DIRECTION('ref_axis',(0.,0.,1.));
#31384=DIRECTION('center_axis',(6.19544098563146E-17,1.,0.));
#31385=DIRECTION('ref_axis',(-1.,6.19544098563145E-17,0.));
#31386=DIRECTION('center_axis',(-0.707106781186525,0.70710678118657,-5.58970135504356E-14));
#31387=DIRECTION('ref_axis',(0.70710678118657,0.707106781186525,-2.27753512105411E-11));
#31388=DIRECTION('center_axis',(0.,1.,0.));
#31389=DIRECTION('ref_axis',(0.,0.,1.));
#31390=DIRECTION('center_axis',(-0.707106781186534,0.707106781186561,3.09217521768369E-14));
#31391=DIRECTION('ref_axis',(0.707106781186561,0.707106781186534,4.69170049623784E-11));
#31392=DIRECTION('center_axis',(6.19544098563146E-17,1.,0.));
#31393=DIRECTION('ref_axis',(-1.,6.19544098563145E-17,0.));
#31394=DIRECTION('',(0.,1.,0.));
#31395=DIRECTION('center_axis',(0.,1.,0.));
#31396=DIRECTION('ref_axis',(0.,0.,1.));
#31397=DIRECTION('center_axis',(6.19544098563146E-17,1.,0.));
#31398=DIRECTION('ref_axis',(-1.,6.19544098563145E-17,0.));
#31399=DIRECTION('center_axis',(0.707106781186567,0.707106781186528,-3.8057541140834E-14));
#31400=DIRECTION('ref_axis',(0.707106781186528,-0.707106781186567,-3.28609365367872E-11));
#31401=DIRECTION('center_axis',(0.,1.,0.));
#31402=DIRECTION('ref_axis',(0.,0.,1.));
#31403=DIRECTION('center_axis',(0.707106781186564,0.707106781186531,3.3300348498065E-14));
#31404=DIRECTION('ref_axis',(0.707106781186531,-0.707106781186564,-8.01952541386524E-13));
#31405=DIRECTION('center_axis',(-0.707106781186544,0.707106781186551,0.));
#31406=DIRECTION('ref_axis',(-0.707106781186551,-0.707106781186544,0.));
#31407=DIRECTION('',(0.,0.,1.));
#31408=DIRECTION('',(0.,0.,1.));
#31409=DIRECTION('',(-0.707106781186551,-0.707106781186544,0.));
#31410=DIRECTION('center_axis',(6.19544098563146E-17,1.,0.));
#31411=DIRECTION('ref_axis',(-1.,6.19544098563146E-17,0.));
#31412=DIRECTION('',(0.,0.,1.));
#31413=DIRECTION('',(0.,0.,1.));
#31414=DIRECTION('center_axis',(0.707106781186551,0.707106781186544,0.));
#31415=DIRECTION('ref_axis',(-0.707106781186544,0.707106781186551,0.));
#31416=DIRECTION('',(0.,0.,1.));
#31417=DIRECTION('center_axis',(1.22464679914735E-16,-1.,0.));
#31418=DIRECTION('ref_axis',(1.,1.22464679914735E-16,0.));
#31419=DIRECTION('',(0.,0.,1.));
#31420=DIRECTION('',(0.,0.,1.));
#31421=DIRECTION('',(0.,0.,1.));
#31422=DIRECTION('',(0.,0.,1.));
#31423=DIRECTION('',(0.,0.,1.));
#31424=DIRECTION('',(0.,0.,1.));
#31425=DIRECTION('',(0.,0.,1.));
#31426=DIRECTION('',(0.,0.,1.));
#31427=DIRECTION('',(1.,1.22464679914735E-16,0.));
#31428=DIRECTION('',(0.,0.,1.));
#31429=DIRECTION('',(1.,1.22464679914735E-16,0.));
#31430=DIRECTION('center_axis',(1.22464679914735E-16,-1.,0.));
#31431=DIRECTION('ref_axis',(1.,1.22464679914735E-16,0.));
#31432=DIRECTION('',(0.,0.,1.));
#31433=DIRECTION('',(1.,1.22464679914735E-16,0.));
#31434=DIRECTION('',(0.,0.,1.));
#31435=DIRECTION('',(1.,1.22464679914735E-16,0.));
#31436=DIRECTION('',(0.,0.,1.));
#31437=DIRECTION('',(0.,0.,1.));
#31438=DIRECTION('',(0.,0.,1.));
#31439=DIRECTION('',(0.,0.,1.));
#31440=DIRECTION('',(0.,0.,1.));
#31441=DIRECTION('',(0.,0.,1.));
#31442=DIRECTION('',(0.,0.,1.));
#31443=DIRECTION('center_axis',(-0.707106781186544,0.707106781186551,0.));
#31444=DIRECTION('ref_axis',(-0.707106781186551,-0.707106781186544,0.));
#31445=DIRECTION('center_axis',(6.19544098563146E-17,1.,0.));
#31446=DIRECTION('ref_axis',(-1.,6.19544098563146E-17,0.));
#31447=DIRECTION('',(0.,0.,1.));
#31448=DIRECTION('',(0.,0.,1.));
#31449=DIRECTION('center_axis',(0.707106781186551,0.707106781186544,0.));
#31450=DIRECTION('ref_axis',(-0.707106781186544,0.707106781186551,0.));
#31451=DIRECTION('center_axis',(-0.707106781186544,0.707106781186551,0.));
#31452=DIRECTION('ref_axis',(-0.707106781186551,-0.707106781186544,0.));
#31453=DIRECTION('center_axis',(6.19544098563146E-17,1.,0.));
#31454=DIRECTION('ref_axis',(-1.,6.19544098563146E-17,0.));
#31455=DIRECTION('',(0.,0.,1.));
#31456=DIRECTION('',(0.,0.,1.));
#31457=DIRECTION('center_axis',(0.707106781186551,0.707106781186544,0.));
#31458=DIRECTION('ref_axis',(-0.707106781186544,0.707106781186551,0.));
#31459=DIRECTION('center_axis',(-0.707106781186544,0.707106781186551,0.));
#31460=DIRECTION('ref_axis',(-0.707106781186551,-0.707106781186544,0.));
#31461=DIRECTION('center_axis',(0.707106781186551,0.707106781186544,0.));
#31462=DIRECTION('ref_axis',(-0.707106781186544,0.707106781186551,0.));
#31463=DIRECTION('',(0.,0.,1.));
#31464=DIRECTION('center_axis',(6.19544098563146E-17,1.,0.));
#31465=DIRECTION('ref_axis',(-1.,6.19544098563146E-17,0.));
#31466=DIRECTION('',(0.,0.,1.));
#31467=DIRECTION('center_axis',(-0.707106781186544,0.707106781186551,0.));
#31468=DIRECTION('ref_axis',(-0.707106781186551,-0.707106781186544,0.));
#31469=DIRECTION('center_axis',(6.19544098563146E-17,1.,0.));
#31470=DIRECTION('ref_axis',(-1.,6.19544098563146E-17,0.));
#31471=DIRECTION('',(0.,0.,1.));
#31472=DIRECTION('',(0.,0.,1.));
#31473=DIRECTION('center_axis',(0.707106781186551,0.707106781186544,0.));
#31474=DIRECTION('ref_axis',(-0.707106781186544,0.707106781186551,0.));
#31475=DIRECTION('center_axis',(-0.707106781186544,0.707106781186551,0.));
#31476=DIRECTION('ref_axis',(-0.707106781186551,-0.707106781186544,0.));
#31477=DIRECTION('center_axis',(6.19544098563146E-17,1.,0.));
#31478=DIRECTION('ref_axis',(-1.,6.19544098563146E-17,0.));
#31479=DIRECTION('',(0.,0.,1.));
#31480=DIRECTION('',(0.,0.,1.));
#31481=DIRECTION('center_axis',(0.707106781186551,0.707106781186544,0.));
#31482=DIRECTION('ref_axis',(-0.707106781186544,0.707106781186551,0.));
#31483=DIRECTION('center_axis',(-0.707106781186544,0.707106781186551,0.));
#31484=DIRECTION('ref_axis',(-0.707106781186551,-0.707106781186544,0.));
#31485=DIRECTION('center_axis',(6.19544098563146E-17,1.,0.));
#31486=DIRECTION('ref_axis',(-1.,6.19544098563146E-17,0.));
#31487=DIRECTION('',(0.,0.,1.));
#31488=DIRECTION('',(0.,0.,1.));
#31489=DIRECTION('center_axis',(0.707106781186551,0.707106781186544,0.));
#31490=DIRECTION('ref_axis',(-0.707106781186544,0.707106781186551,0.));
#31491=DIRECTION('center_axis',(-0.707106781186544,0.707106781186551,0.));
#31492=DIRECTION('ref_axis',(-0.707106781186551,-0.707106781186544,0.));
#31493=DIRECTION('center_axis',(6.19544098563146E-17,1.,0.));
#31494=DIRECTION('ref_axis',(-1.,6.19544098563146E-17,0.));
#31495=DIRECTION('',(0.,0.,1.));
#31496=DIRECTION('',(0.,0.,1.));
#31497=DIRECTION('',(-1.,6.19544098563146E-17,0.));
#31498=DIRECTION('center_axis',(0.707106781186551,0.707106781186544,0.));
#31499=DIRECTION('ref_axis',(-0.707106781186544,0.707106781186551,0.));
#31500=DIRECTION('',(-0.707106781186544,0.707106781186551,0.));
#31501=DIRECTION('center_axis',(0.,0.,-1.));
#31502=DIRECTION('ref_axis',(-1.,0.,0.));
#31503=DIRECTION('',(0.707106781186544,-0.707106781186551,0.));
#31504=DIRECTION('',(0.,-1.,0.));
#31505=DIRECTION('center_axis',(0.,0.,-1.));
#31506=DIRECTION('ref_axis',(-1.,0.,0.));
#31507=DIRECTION('',(-0.707106781186551,-0.707106781186544,0.));
#31508=DIRECTION('center_axis',(0.,0.,1.));
#31509=DIRECTION('ref_axis',(-1.,0.,0.));
#31510=DIRECTION('',(0.,-1.,0.));
#31511=DIRECTION('center_axis',(0.,0.,1.));
#31512=DIRECTION('ref_axis',(-1.,0.,0.));
#31513=DIRECTION('',(0.707106781186544,-0.707106781186551,0.));
#31514=DIRECTION('center_axis',(0.,0.,-1.));
#31515=DIRECTION('ref_axis',(-1.,0.,0.));
#31516=DIRECTION('center_axis',(0.,0.,1.));
#31517=DIRECTION('ref_axis',(1.,0.,0.));
#31518=DIRECTION('center_axis',(0.,0.,-1.));
#31519=DIRECTION('ref_axis',(-1.,0.,0.));
#31520=DIRECTION('',(0.707106781186544,-0.707106781186551,0.));
#31521=DIRECTION('center_axis',(0.,0.,-1.));
#31522=DIRECTION('ref_axis',(-1.,0.,0.));
#31523=DIRECTION('',(0.,-1.,0.));
#31524=DIRECTION('center_axis',(0.,0.,-1.));
#31525=DIRECTION('ref_axis',(-1.,0.,0.));
#31526=DIRECTION('',(-0.70710678118655,-0.707106781186545,0.));
#31527=DIRECTION('center_axis',(0.,0.,-1.));
#31528=DIRECTION('ref_axis',(-1.,0.,0.));
#31529=DIRECTION('center_axis',(0.,0.,1.));
#31530=DIRECTION('ref_axis',(1.,0.,0.));
#31531=DIRECTION('center_axis',(0.,0.,-1.));
#31532=DIRECTION('ref_axis',(-1.,0.,0.));
#31533=DIRECTION('',(-0.70710678118655,-0.707106781186545,0.));
#31534=DIRECTION('',(-1.,0.,0.));
#31535=DIRECTION('',(0.70710678118655,-0.707106781186545,0.));
#31536=DIRECTION('center_axis',(0.,0.,-1.));
#31537=DIRECTION('ref_axis',(-1.,0.,0.));
#31538=DIRECTION('center_axis',(0.,0.,-1.));
#31539=DIRECTION('ref_axis',(-1.,0.,0.));
#31540=DIRECTION('center_axis',(0.,0.,-1.));
#31541=DIRECTION('ref_axis',(-1.,0.,0.));
#31542=DIRECTION('',(0.70710678118655,-0.707106781186545,0.));
#31543=DIRECTION('center_axis',(0.,0.,-1.));
#31544=DIRECTION('ref_axis',(-1.,0.,0.));
#31545=DIRECTION('',(0.,-1.,0.));
#31546=DIRECTION('center_axis',(0.,0.,-1.));
#31547=DIRECTION('ref_axis',(-1.,0.,0.));
#31548=DIRECTION('',(-0.707106781186544,-0.707106781186551,0.));
#31549=DIRECTION('center_axis',(0.,0.,-1.));
#31550=DIRECTION('ref_axis',(-1.,0.,0.));
#31551=DIRECTION('center_axis',(0.,0.,-1.));
#31552=DIRECTION('ref_axis',(-1.,0.,0.));
#31553=DIRECTION('center_axis',(0.,0.,-1.));
#31554=DIRECTION('ref_axis',(-1.,0.,0.));
#31555=DIRECTION('',(-0.707106781186544,-0.707106781186551,0.));
#31556=DIRECTION('center_axis',(0.,0.,1.));
#31557=DIRECTION('ref_axis',(-1.,-3.46944695195361E-15,0.));
#31558=DIRECTION('',(0.,-1.,0.));
#31559=DIRECTION('center_axis',(0.,0.,1.));
#31560=DIRECTION('ref_axis',(-1.,0.,0.));
#31561=DIRECTION('',(0.707106781186551,-0.707106781186544,0.));
#31562=DIRECTION('center_axis',(0.,0.,-1.));
#31563=DIRECTION('ref_axis',(-1.,0.,0.));
#31564=DIRECTION('',(0.,-1.,0.));
#31565=DIRECTION('',(-0.707106781186544,-0.707106781186551,0.));
#31566=DIRECTION('',(-0.707106781186544,0.707106781186551,0.));
#31567=DIRECTION('',(-1.,6.19544098563146E-17,0.));
#31568=DIRECTION('center_axis',(0.,0.,-1.));
#31569=DIRECTION('ref_axis',(-1.,0.,0.));
#31570=DIRECTION('',(-0.707106781186551,-0.707106781186544,0.));
#31571=DIRECTION('',(-0.707106781186544,-0.707106781186551,0.));
#31572=DIRECTION('',(0.,-1.,0.));
#31573=DIRECTION('center_axis',(0.,0.,1.));
#31574=DIRECTION('ref_axis',(-1.,1.73472347597681E-15,0.));
#31575=DIRECTION('',(0.707106781186551,-0.707106781186544,0.));
#31576=DIRECTION('center_axis',(0.,0.,-1.));
#31577=DIRECTION('ref_axis',(-1.,0.,0.));
#31578=DIRECTION('',(0.,-1.,0.));
#31579=DIRECTION('center_axis',(0.,0.,-1.));
#31580=DIRECTION('ref_axis',(-1.,0.,0.));
#31581=DIRECTION('',(-0.707106781186544,-0.707106781186551,0.));
#31582=DIRECTION('center_axis',(0.,0.,1.));
#31583=DIRECTION('ref_axis',(-1.,0.,0.));
#31584=DIRECTION('center_axis',(0.,0.,-1.));
#31585=DIRECTION('ref_axis',(-1.,0.,0.));
#31586=DIRECTION('center_axis',(0.,0.,1.));
#31587=DIRECTION('ref_axis',(-1.,-6.93889390390722E-15,0.));
#31588=DIRECTION('',(-0.707106781186544,-0.707106781186551,0.));
#31589=DIRECTION('center_axis',(0.,0.,1.));
#31590=DIRECTION('ref_axis',(-1.,0.,0.));
#31591=DIRECTION('',(0.,-1.,0.));
#31592=DIRECTION('center_axis',(0.,0.,1.));
#31593=DIRECTION('ref_axis',(-1.,0.,0.));
#31594=DIRECTION('',(0.70710678118655,-0.707106781186545,0.));
#31595=DIRECTION('center_axis',(0.,0.,1.));
#31596=DIRECTION('ref_axis',(-1.,0.,0.));
#31597=DIRECTION('center_axis',(0.,0.,-1.));
#31598=DIRECTION('ref_axis',(-1.,0.,0.));
#31599=DIRECTION('center_axis',(0.,0.,1.));
#31600=DIRECTION('ref_axis',(-1.,0.,0.));
#31601=DIRECTION('',(0.70710678118655,-0.707106781186545,0.));
#31602=DIRECTION('',(-1.,0.,0.));
#31603=DIRECTION('',(-0.70710678118655,-0.707106781186545,0.));
#31604=DIRECTION('center_axis',(0.,0.,1.));
#31605=DIRECTION('ref_axis',(-1.,0.,0.));
#31606=DIRECTION('center_axis',(0.,0.,1.));
#31607=DIRECTION('ref_axis',(1.,0.,0.));
#31608=DIRECTION('center_axis',(0.,0.,1.));
#31609=DIRECTION('ref_axis',(-1.,-6.93889390390722E-15,0.));
#31610=DIRECTION('',(-0.70710678118655,-0.707106781186545,0.));
#31611=DIRECTION('center_axis',(0.,0.,1.));
#31612=DIRECTION('ref_axis',(-1.,6.93889390390722E-15,0.));
#31613=DIRECTION('',(0.,-1.,0.));
#31614=DIRECTION('center_axis',(0.,0.,1.));
#31615=DIRECTION('ref_axis',(-1.,0.,0.));
#31616=DIRECTION('',(0.707106781186544,-0.707106781186551,0.));
#31617=DIRECTION('center_axis',(0.,0.,1.));
#31618=DIRECTION('ref_axis',(-1.,0.,0.));
#31619=DIRECTION('center_axis',(0.,0.,1.));
#31620=DIRECTION('ref_axis',(1.,0.,0.));
#31621=DIRECTION('center_axis',(0.,0.,1.));
#31622=DIRECTION('ref_axis',(-1.,0.,0.));
#31623=DIRECTION('',(0.707106781186544,-0.707106781186551,0.));
#31624=DIRECTION('center_axis',(0.,0.,-1.));
#31625=DIRECTION('ref_axis',(-1.,0.,0.));
#31626=DIRECTION('',(0.,-1.,0.));
#31627=DIRECTION('center_axis',(0.,0.,-1.));
#31628=DIRECTION('ref_axis',(-1.,0.,0.));
#31629=DIRECTION('',(-0.707106781186551,-0.707106781186544,0.));
#31630=DIRECTION('center_axis',(0.,0.,1.));
#31631=DIRECTION('ref_axis',(-1.,1.12757025938493E-14,0.));
#31632=DIRECTION('',(0.,-1.,0.));
#31633=DIRECTION('',(0.707106781186544,-0.707106781186551,0.));
#31634=DIRECTION('center_axis',(-0.707106781186551,0.707106781186544,0.));
#31635=DIRECTION('ref_axis',(-0.707106781186544,-0.707106781186551,0.));
#31636=DIRECTION('',(0.,0.,-1.));
#31637=DIRECTION('',(0.,0.,1.));
#31638=DIRECTION('center_axis',(-0.707106781186551,0.707106781186544,0.));
#31639=DIRECTION('ref_axis',(-0.707106781186544,-0.707106781186551,0.));
#31640=DIRECTION('',(0.,0.,1.));
#31641=DIRECTION('',(0.,0.,-1.));
#31642=DIRECTION('center_axis',(-0.707106781186545,-0.70710678118655,0.));
#31643=DIRECTION('ref_axis',(0.70710678118655,-0.707106781186545,0.));
#31644=DIRECTION('',(0.,0.,1.));
#31645=DIRECTION('',(0.,0.,-1.));
#31646=DIRECTION('center_axis',(-0.707106781186545,-0.70710678118655,0.));
#31647=DIRECTION('ref_axis',(0.70710678118655,-0.707106781186545,0.));
#31648=DIRECTION('',(0.,0.,-1.));
#31649=DIRECTION('',(0.,0.,1.));
#31650=DIRECTION('center_axis',(-0.707106781186551,-0.707106781186544,0.));
#31651=DIRECTION('ref_axis',(0.707106781186544,-0.707106781186551,0.));
#31652=DIRECTION('',(0.,0.,1.));
#31653=DIRECTION('',(0.,0.,-1.));
#31654=DIRECTION('center_axis',(-0.707106781186545,0.70710678118655,0.));
#31655=DIRECTION('ref_axis',(-0.70710678118655,-0.707106781186545,0.));
#31656=DIRECTION('',(0.,0.,-1.));
#31657=DIRECTION('',(0.,0.,1.));
#31658=DIRECTION('center_axis',(0.,1.,0.));
#31659=DIRECTION('ref_axis',(0.,0.,1.));
#31660=DIRECTION('',(0.,0.,1.));
#31661=DIRECTION('center_axis',(-0.707106781186551,-0.707106781186544,0.));
#31662=DIRECTION('ref_axis',(0.707106781186544,-0.707106781186551,0.));
#31663=DIRECTION('',(0.,0.,1.));
#31664=DIRECTION('center_axis',(-1.,0.,0.));
#31665=DIRECTION('ref_axis',(0.,0.,1.));
#31666=DIRECTION('',(0.,0.,-1.));
#31667=DIRECTION('center_axis',(-0.707106781186544,0.707106781186551,0.));
#31668=DIRECTION('ref_axis',(-0.707106781186551,-0.707106781186544,0.));
#31669=DIRECTION('',(0.,0.,1.));
#31670=DIRECTION('',(0.,0.,-1.));
#31671=DIRECTION('center_axis',(-1.,0.,0.));
#31672=DIRECTION('ref_axis',(0.,0.,1.));
#31673=DIRECTION('',(0.,0.,1.));
#31674=DIRECTION('',(0.,0.,-1.));
#31675=DIRECTION('center_axis',(-0.707106781186551,-0.707106781186544,0.));
#31676=DIRECTION('ref_axis',(0.707106781186544,-0.707106781186551,0.));
#31677=DIRECTION('',(0.,0.,-1.));
#31678=DIRECTION('',(0.,0.,1.));
#31679=DIRECTION('center_axis',(-1.,0.,0.));
#31680=DIRECTION('ref_axis',(0.,0.,1.));
#31681=DIRECTION('',(0.,0.,-1.));
#31682=DIRECTION('',(0.,0.,1.));
#31683=DIRECTION('center_axis',(-0.707106781186545,0.70710678118655,0.));
#31684=DIRECTION('ref_axis',(-0.70710678118655,-0.707106781186545,0.));
#31685=DIRECTION('',(0.,0.,1.));
#31686=DIRECTION('center_axis',(0.,0.,1.));
#31687=DIRECTION('ref_axis',(1.,0.,0.));
#31688=DIRECTION('',(0.,0.,1.));
#31689=DIRECTION('',(0.,0.,-1.));
#31690=DIRECTION('center_axis',(0.,0.,1.));
#31691=DIRECTION('ref_axis',(1.,0.,0.));
#31692=DIRECTION('',(0.,0.,-1.));
#31693=DIRECTION('',(0.,0.,1.));
#31694=DIRECTION('center_axis',(0.,0.,1.));
#31695=DIRECTION('ref_axis',(1.,0.,0.));
#31696=DIRECTION('center_axis',(0.,0.,1.));
#31697=DIRECTION('ref_axis',(1.,0.,0.));
#31698=DIRECTION('center_axis',(0.,0.,1.));
#31699=DIRECTION('ref_axis',(1.,0.,0.));
#31700=DIRECTION('center_axis',(0.,0.,1.));
#31701=DIRECTION('ref_axis',(1.,0.,0.));
#31702=DIRECTION('center_axis',(0.,0.,-1.));
#31703=DIRECTION('ref_axis',(-1.,0.,0.));
#31704=DIRECTION('center_axis',(0.,0.,-1.));
#31705=DIRECTION('ref_axis',(-1.,0.,0.));
#31706=DIRECTION('center_axis',(0.,0.,1.));
#31707=DIRECTION('ref_axis',(1.,0.,0.));
#31708=DIRECTION('center_axis',(0.,0.,1.));
#31709=DIRECTION('ref_axis',(1.,0.,0.));
#31710=DIRECTION('center_axis',(0.,0.,1.));
#31711=DIRECTION('ref_axis',(1.,0.,0.));
#31712=DIRECTION('center_axis',(-1.,0.,0.));
#31713=DIRECTION('ref_axis',(0.,0.,1.));
#31714=DIRECTION('',(0.,0.,1.));
#31715=DIRECTION('',(0.,0.,-1.));
#31716=DIRECTION('center_axis',(-1.,0.,0.));
#31717=DIRECTION('ref_axis',(0.,0.,1.));
#31718=DIRECTION('',(0.,0.,-1.));
#31719=DIRECTION('',(0.,0.,1.));
#31720=DIRECTION('center_axis',(-0.707106781186544,-0.707106781186551,0.));
#31721=DIRECTION('ref_axis',(0.707106781186551,-0.707106781186544,0.));
#31722=DIRECTION('',(0.,0.,-1.));
#31723=DIRECTION('',(0.,0.,1.));
#31724=DIRECTION('center_axis',(-1.,0.,0.));
#31725=DIRECTION('ref_axis',(0.,0.,1.));
#31726=DIRECTION('',(0.,0.,1.));
#31727=DIRECTION('',(0.,0.,1.));
#31728=DIRECTION('center_axis',(-0.707106781186551,0.707106781186544,0.));
#31729=DIRECTION('ref_axis',(-0.707106781186544,-0.707106781186551,0.));
#31730=DIRECTION('center_axis',(0.,0.,1.));
#31731=DIRECTION('ref_axis',(1.,0.,0.));
#31732=DIRECTION('',(0.,0.,-1.));
#31733=DIRECTION('',(0.,0.,1.));
#31734=DIRECTION('center_axis',(0.,0.,1.));
#31735=DIRECTION('ref_axis',(1.,0.,0.));
#31736=DIRECTION('',(0.,0.,1.));
#31737=DIRECTION('',(0.,0.,-1.));
#31738=DIRECTION('center_axis',(0.,0.,1.));
#31739=DIRECTION('ref_axis',(1.,0.,0.));
#31740=DIRECTION('center_axis',(0.,0.,1.));
#31741=DIRECTION('ref_axis',(1.,0.,0.));
#31742=DIRECTION('center_axis',(0.,0.,1.));
#31743=DIRECTION('ref_axis',(1.,0.,0.));
#31744=DIRECTION('center_axis',(0.,0.,1.));
#31745=DIRECTION('ref_axis',(1.,0.,0.));
#31746=DIRECTION('center_axis',(0.,0.,-1.));
#31747=DIRECTION('ref_axis',(-1.,0.,0.));
#31748=DIRECTION('center_axis',(0.,0.,-1.));
#31749=DIRECTION('ref_axis',(-1.,0.,0.));
#31750=DIRECTION('center_axis',(0.,0.,1.));
#31751=DIRECTION('ref_axis',(1.,0.,0.));
#31752=DIRECTION('center_axis',(0.,0.,1.));
#31753=DIRECTION('ref_axis',(1.,0.,0.));
#31754=DIRECTION('center_axis',(0.,0.,1.));
#31755=DIRECTION('ref_axis',(1.,0.,0.));
#31756=DIRECTION('center_axis',(-0.707106781186544,0.707106781186551,0.));
#31757=DIRECTION('ref_axis',(-0.707106781186551,-0.707106781186544,0.));
#31758=DIRECTION('center_axis',(6.19544098563146E-17,1.,0.));
#31759=DIRECTION('ref_axis',(-1.,6.19544098563146E-17,0.));
#31760=DIRECTION('',(0.,0.,1.));
#31761=DIRECTION('center_axis',(0.707106781186551,0.707106781186544,0.));
#31762=DIRECTION('ref_axis',(-0.707106781186544,0.707106781186551,0.));
#31763=DIRECTION('center_axis',(0.,-1.,0.));
#31764=DIRECTION('ref_axis',(0.,0.,-1.));
#31765=DIRECTION('center_axis',(0.,-1.,0.));
#31766=DIRECTION('ref_axis',(0.,0.,-1.));
#31767=DIRECTION('center_axis',(0.,-1.,0.));
#31768=DIRECTION('ref_axis',(0.,0.,-1.));
#31769=DIRECTION('center_axis',(0.,-1.,0.));
#31770=DIRECTION('ref_axis',(0.,0.,-1.));
#31771=DIRECTION('center_axis',(0.,-1.,0.));
#31772=DIRECTION('ref_axis',(0.,0.,-1.));
#31773=DIRECTION('center_axis',(0.,-1.,0.));
#31774=DIRECTION('ref_axis',(0.,0.,-1.));
#31775=DIRECTION('center_axis',(0.,-1.,0.));
#31776=DIRECTION('ref_axis',(0.,0.,-1.));
#31777=DIRECTION('center_axis',(0.,-1.,0.));
#31778=DIRECTION('ref_axis',(0.,0.,-1.));
#53469=CARTESIAN_POINT('',(0.,0.,0.));
#53470=CARTESIAN_POINT('Origin',(0.,22.,-420.));
#53471=CARTESIAN_POINT('',(-6.73555739531045E-16,13.,-425.5));
#53472=CARTESIAN_POINT('Origin',(0.,13.,-420.));
#53473=CARTESIAN_POINT('',(-6.73555739531045E-16,22.,-425.5));
#53474=CARTESIAN_POINT('',(-6.73555739531045E-16,22.,-425.5));
#53475=CARTESIAN_POINT('Origin',(0.,22.,-420.));
#53476=CARTESIAN_POINT('Origin',(0.,22.,-420.));
#53477=CARTESIAN_POINT('',(-1.75,0.500000000000001,-416.968911086754));
#53478=CARTESIAN_POINT('',(1.75,0.5,-416.968911086754));
#53479=CARTESIAN_POINT('Origin',(0.,0.5,-420.));
#53480=CARTESIAN_POINT('',(-2.25,0.,-417.319048676309));
#53481=CARTESIAN_POINT('Origin',(1.23513471672609E-8,2.25000001235081,-420.000000017303));
#53482=CARTESIAN_POINT('',(-2.25,0.,-422.680951323691));
#53483=CARTESIAN_POINT('Origin',(0.,0.,-420.));
#53484=CARTESIAN_POINT('',(-1.75,0.500000000000001,-423.031088913246));
#53485=CARTESIAN_POINT('Origin',(-3.10164607886243E-8,2.24999996898292,
-420.000000044163));
#53486=CARTESIAN_POINT('',(-4.28626379701572E-16,0.499999999999998,-423.5));
#53487=CARTESIAN_POINT('Origin',(0.,0.5,-420.));
#53488=CARTESIAN_POINT('',(-4.28626379701574E-16,13.,-423.5));
#53489=CARTESIAN_POINT('',(-4.28626379701574E-16,22.,-423.5));
#53490=CARTESIAN_POINT('Origin',(0.,13.,-420.));
#53491=CARTESIAN_POINT('',(1.75,0.5,-423.031088913246));
#53492=CARTESIAN_POINT('Origin',(0.,0.5,-420.));
#53493=CARTESIAN_POINT('',(2.25,0.,-422.680951323691));
#53494=CARTESIAN_POINT('Origin',(-2.43443196157322E-8,2.25000002434478,
-419.999999965121));
#53495=CARTESIAN_POINT('',(2.25,0.,-417.319048676309));
#53496=CARTESIAN_POINT('Origin',(0.,0.,-420.));
#53497=CARTESIAN_POINT('Origin',(1.14266326955992E-8,2.24999998857398,-419.999999982967));
#53498=CARTESIAN_POINT('Origin',(0.,22.,-360.));
#53499=CARTESIAN_POINT('',(-6.73555739531045E-16,13.,-365.5));
#53500=CARTESIAN_POINT('Origin',(0.,13.,-360.));
#53501=CARTESIAN_POINT('',(-6.73555739531045E-16,22.,-365.5));
#53502=CARTESIAN_POINT('',(-6.73555739531045E-16,22.,-365.5));
#53503=CARTESIAN_POINT('Origin',(0.,22.,-360.));
#53504=CARTESIAN_POINT('Origin',(0.,22.,-360.));
#53505=CARTESIAN_POINT('',(-1.75,0.500000000000001,-356.968911086754));
#53506=CARTESIAN_POINT('',(1.75,0.5,-356.968911086754));
#53507=CARTESIAN_POINT('Origin',(0.,0.5,-360.));
#53508=CARTESIAN_POINT('',(-2.25,0.,-357.319048676309));
#53509=CARTESIAN_POINT('Origin',(-1.81638087903835E-8,2.24999998183567,
-359.999999973801));
#53510=CARTESIAN_POINT('',(-2.25,0.,-362.680951323691));
#53511=CARTESIAN_POINT('Origin',(0.,0.,-360.));
#53512=CARTESIAN_POINT('',(-1.75,0.500000000000001,-363.031088913246));
#53513=CARTESIAN_POINT('Origin',(-4.23829027429434E-10,2.24999999957564,
-360.000000000522));
#53514=CARTESIAN_POINT('',(-4.28626379701572E-16,0.499999999999998,-363.5));
#53515=CARTESIAN_POINT('Origin',(0.,0.5,-360.));
#53516=CARTESIAN_POINT('',(-4.28626379701574E-16,13.,-363.5));
#53517=CARTESIAN_POINT('',(-4.28626379701574E-16,22.,-363.5));
#53518=CARTESIAN_POINT('Origin',(0.,13.,-360.));
#53519=CARTESIAN_POINT('',(1.75,0.5,-363.031088913246));
#53520=CARTESIAN_POINT('Origin',(0.,0.5,-360.));
#53521=CARTESIAN_POINT('',(2.24999999999999,0.,-362.680951323691));
#53522=CARTESIAN_POINT('Origin',(-1.81887060968222E-9,2.25000000181898,
-359.99999999671));
#53523=CARTESIAN_POINT('',(2.24999999999999,0.,-357.319048676309));
#53524=CARTESIAN_POINT('Origin',(0.,0.,-360.));
#53525=CARTESIAN_POINT('Origin',(-4.00230404373758E-8,2.2500000400232,-360.000000056605));
#53526=CARTESIAN_POINT('Origin',(0.,22.,-300.));
#53527=CARTESIAN_POINT('',(-6.73555739531045E-16,13.,-305.5));
#53528=CARTESIAN_POINT('Origin',(0.,13.,-300.));
#53529=CARTESIAN_POINT('',(-6.73555739531045E-16,22.,-305.5));
#53530=CARTESIAN_POINT('',(-6.73555739531045E-16,22.,-305.5));
#53531=CARTESIAN_POINT('Origin',(0.,22.,-300.));
#53532=CARTESIAN_POINT('Origin',(0.,22.,-300.));
#53533=CARTESIAN_POINT('',(-1.75,0.500000000000001,-296.968911086754));
#53534=CARTESIAN_POINT('',(1.75,0.5,-296.968911086754));
#53535=CARTESIAN_POINT('Origin',(0.,0.5,-300.));
#53536=CARTESIAN_POINT('',(-2.25,0.,-297.319048676309));
#53537=CARTESIAN_POINT('Origin',(-6.9596634011404E-10,2.24999999930352,
-299.999999999323));
#53538=CARTESIAN_POINT('',(-2.25,0.,-302.680951323691));
#53539=CARTESIAN_POINT('Origin',(0.,0.,-300.));
#53540=CARTESIAN_POINT('',(-1.75,0.500000000000001,-303.031088913246));
#53541=CARTESIAN_POINT('Origin',(-5.11468117858627E-9,2.24999999488474,
-300.000000007122));
#53542=CARTESIAN_POINT('',(-4.28626379701572E-16,0.499999999999998,-303.5));
#53543=CARTESIAN_POINT('Origin',(0.,0.5,-300.));
#53544=CARTESIAN_POINT('',(-4.28626379701574E-16,13.,-303.5));
#53545=CARTESIAN_POINT('',(-4.28626379701574E-16,22.,-303.5));
#53546=CARTESIAN_POINT('Origin',(0.,13.,-300.));
#53547=CARTESIAN_POINT('',(1.75,0.5,-303.031088913246));
#53548=CARTESIAN_POINT('Origin',(0.,0.5,-300.));
#53549=CARTESIAN_POINT('',(2.24999999999999,0.,-302.680951323691));
#53550=CARTESIAN_POINT('Origin',(1.1544250833051E-8,2.24999998845594,-300.000000016304));
#53551=CARTESIAN_POINT('',(2.24999999999999,0.,-297.319048676309));
#53552=CARTESIAN_POINT('Origin',(0.,0.,-300.));
#53553=CARTESIAN_POINT('Origin',(4.10078357382382E-8,2.2499999589923,-299.999999941256));
#53554=CARTESIAN_POINT('Origin',(0.,22.,-240.));
#53555=CARTESIAN_POINT('',(-6.73555739531045E-16,13.,-245.5));
#53556=CARTESIAN_POINT('Origin',(0.,13.,-240.));
#53557=CARTESIAN_POINT('',(-6.73555739531045E-16,22.,-245.5));
#53558=CARTESIAN_POINT('',(-6.73555739531045E-16,22.,-245.5));
#53559=CARTESIAN_POINT('Origin',(0.,22.,-240.));
#53560=CARTESIAN_POINT('Origin',(0.,22.,-240.));
#53561=CARTESIAN_POINT('',(-1.75,0.500000000000001,-236.968911086754));
#53562=CARTESIAN_POINT('',(1.75,0.5,-236.968911086754));
#53563=CARTESIAN_POINT('Origin',(0.,0.5,-240.));
#53564=CARTESIAN_POINT('',(-2.25,0.,-237.319048676309));
#53565=CARTESIAN_POINT('Origin',(2.09455894295552E-8,2.25000002094498,-240.00000002998));
#53566=CARTESIAN_POINT('',(-2.25,0.,-242.680951323691));
#53567=CARTESIAN_POINT('Origin',(0.,0.,-240.));
#53568=CARTESIAN_POINT('',(-1.75,0.500000000000001,-243.031088913246));
#53569=CARTESIAN_POINT('Origin',(-3.71720848546531E-9,2.24999999628211,
-240.000000004996));
#53570=CARTESIAN_POINT('',(-4.28626379701572E-16,0.499999999999998,-243.5));
#53571=CARTESIAN_POINT('Origin',(0.,0.5,-240.));
#53572=CARTESIAN_POINT('',(-4.28626379701574E-16,13.,-243.5));
#53573=CARTESIAN_POINT('',(-4.28626379701574E-16,22.,-243.5));
#53574=CARTESIAN_POINT('Origin',(0.,13.,-240.));
#53575=CARTESIAN_POINT('',(1.75,0.5,-243.031088913246));
#53576=CARTESIAN_POINT('Origin',(0.,0.5,-240.));
#53577=CARTESIAN_POINT('',(2.25,0.,-242.680951323691));
#53578=CARTESIAN_POINT('Origin',(-3.97217841952013E-9,2.25000000397282,
-239.999999995265));
#53579=CARTESIAN_POINT('',(2.25,0.,-237.319048676309));
#53580=CARTESIAN_POINT('Origin',(0.,0.,-240.));
#53581=CARTESIAN_POINT('Origin',(9.45980321853668E-9,2.24999999054093,-239.999999986565));
#53582=CARTESIAN_POINT('Origin',(0.,22.,-180.));
#53583=CARTESIAN_POINT('',(-6.73555739531045E-16,13.,-185.5));
#53584=CARTESIAN_POINT('Origin',(0.,13.,-180.));
#53585=CARTESIAN_POINT('',(-6.73555739531045E-16,22.,-185.5));
#53586=CARTESIAN_POINT('',(-6.73555739531045E-16,22.,-185.5));
#53587=CARTESIAN_POINT('Origin',(0.,22.,-180.));
#53588=CARTESIAN_POINT('Origin',(0.,22.,-180.));
#53589=CARTESIAN_POINT('',(-1.75,0.500000000000001,-176.968911086754));
#53590=CARTESIAN_POINT('',(1.75,0.5,-176.968911086755));
#53591=CARTESIAN_POINT('Origin',(0.,0.5,-180.));
#53592=CARTESIAN_POINT('',(-2.25,0.,-177.319048676309));
#53593=CARTESIAN_POINT('Origin',(1.45397632822508E-8,2.25000001453915,-180.000000021041));
#53594=CARTESIAN_POINT('',(-2.25,0.,-182.680951323691));
#53595=CARTESIAN_POINT('Origin',(0.,0.,-180.));
#53596=CARTESIAN_POINT('',(-1.75,0.500000000000001,-183.031088913246));
#53597=CARTESIAN_POINT('Origin',(-1.75473274799387E-9,2.24999999824459,
-180.000000002503));
#53598=CARTESIAN_POINT('',(-4.28626379701572E-16,0.499999999999998,-183.5));
#53599=CARTESIAN_POINT('Origin',(0.,0.5,-180.));
#53600=CARTESIAN_POINT('',(-4.28626379701574E-16,13.,-183.5));
#53601=CARTESIAN_POINT('',(-4.28626379701574E-16,22.,-183.5));
#53602=CARTESIAN_POINT('Origin',(0.,13.,-180.));
#53603=CARTESIAN_POINT('',(1.75,0.5,-183.031088913246));
#53604=CARTESIAN_POINT('Origin',(0.,0.5,-180.));
#53605=CARTESIAN_POINT('',(2.24999999999999,0.,-182.680951323691));
#53606=CARTESIAN_POINT('Origin',(-1.31895855348674E-9,2.25000000131934,
-179.999999998353));
#53607=CARTESIAN_POINT('',(2.24999999999999,0.,-177.319048676309));
#53608=CARTESIAN_POINT('Origin',(0.,0.,-180.));
#53609=CARTESIAN_POINT('Origin',(2.13298301243725E-8,2.24999997867055,-179.999999969452));
#53610=CARTESIAN_POINT('Origin',(0.,22.,-120.));
#53611=CARTESIAN_POINT('',(-6.73555739531045E-16,13.,-125.5));
#53612=CARTESIAN_POINT('Origin',(0.,13.,-120.));
#53613=CARTESIAN_POINT('',(-6.73555739531045E-16,22.,-125.5));
#53614=CARTESIAN_POINT('',(-6.73555739531045E-16,22.,-125.5));
#53615=CARTESIAN_POINT('Origin',(0.,22.,-120.));
#53616=CARTESIAN_POINT('Origin',(0.,22.,-120.));
#53617=CARTESIAN_POINT('',(-1.75,0.500000000000001,-116.968911086754));
#53618=CARTESIAN_POINT('',(1.75,0.5,-116.968911086755));
#53619=CARTESIAN_POINT('Origin',(0.,0.5,-120.));
#53620=CARTESIAN_POINT('',(-2.25,0.,-117.319048676309));
#53621=CARTESIAN_POINT('Origin',(-2.48057657747935E-9,2.24999999751883,
-119.999999996391));
#53622=CARTESIAN_POINT('',(-2.25,0.,-122.680951323691));
#53623=CARTESIAN_POINT('Origin',(0.,0.,-120.));
#53624=CARTESIAN_POINT('',(-1.75,0.500000000000001,-123.031088913246));
#53625=CARTESIAN_POINT('Origin',(6.68797350833472E-9,2.25000000668744,-119.99999999052));
#53626=CARTESIAN_POINT('',(-4.28626379701574E-16,0.499999999999998,-123.5));
#53627=CARTESIAN_POINT('Origin',(0.,0.5,-120.));
#53628=CARTESIAN_POINT('',(-4.28626379701574E-16,13.,-123.5));
#53629=CARTESIAN_POINT('',(-4.28626379701574E-16,22.,-123.5));
#53630=CARTESIAN_POINT('Origin',(0.,13.,-120.));
#53631=CARTESIAN_POINT('',(1.75,0.5,-123.031088913246));
#53632=CARTESIAN_POINT('Origin',(0.,0.5,-120.));
#53633=CARTESIAN_POINT('',(2.24999999999999,0.,-122.680951323691));
#53634=CARTESIAN_POINT('Origin',(-1.15682741164136E-9,2.25000000115695,
-119.999999998469));
#53635=CARTESIAN_POINT('',(2.24999999999999,0.,-117.319048676309));
#53636=CARTESIAN_POINT('Origin',(0.,0.,-120.));
#53637=CARTESIAN_POINT('Origin',(8.38862423968578E-9,2.24999999161153,-119.999999987973));
#53638=CARTESIAN_POINT('Origin',(0.,22.,-60.));
#53639=CARTESIAN_POINT('',(-6.73555739531044E-16,13.,-65.5));
#53640=CARTESIAN_POINT('Origin',(0.,13.,-60.));
#53641=CARTESIAN_POINT('',(-6.73555739531044E-16,22.,-65.5));
#53642=CARTESIAN_POINT('',(-6.73555739531044E-16,22.,-65.5));
#53643=CARTESIAN_POINT('Origin',(0.,22.,-60.));
#53644=CARTESIAN_POINT('Origin',(0.,22.,-60.));
#53645=CARTESIAN_POINT('',(-1.75,0.500000000000001,-56.9689110867545));
#53646=CARTESIAN_POINT('',(1.75,0.5,-56.9689110867546));
#53647=CARTESIAN_POINT('Origin',(0.,0.5,-60.));
#53648=CARTESIAN_POINT('',(-2.25,0.,-57.3190486763091));
#53649=CARTESIAN_POINT('Origin',(-5.2602575073557E-9,2.2499999947395,-59.9999999924325));
#53650=CARTESIAN_POINT('',(-2.25,0.,-62.6809513236909));
#53651=CARTESIAN_POINT('Origin',(0.,0.,-60.));
#53652=CARTESIAN_POINT('',(-1.75,0.500000000000001,-63.0310889132455));
#53653=CARTESIAN_POINT('Origin',(4.60471411001251E-9,2.25000000460459,-59.999999993365));
#53654=CARTESIAN_POINT('',(-4.28626379701573E-16,0.499999999999998,-63.5));
#53655=CARTESIAN_POINT('Origin',(0.,0.5,-60.));
#53656=CARTESIAN_POINT('',(-4.28626379701573E-16,13.,-63.5));
#53657=CARTESIAN_POINT('',(-4.28626379701573E-16,22.,-63.5));
#53658=CARTESIAN_POINT('Origin',(0.,13.,-60.));
#53659=CARTESIAN_POINT('',(1.75,0.5,-63.0310889132457));
#53660=CARTESIAN_POINT('Origin',(0.,0.5,-60.));
#53661=CARTESIAN_POINT('',(2.24999999999999,0.,-62.6809513236909));
#53662=CARTESIAN_POINT('Origin',(-6.26890206412156E-10,2.25000000062714,
-59.9999999992371));
#53663=CARTESIAN_POINT('',(2.24999999999999,0.,-57.3190486763091));
#53664=CARTESIAN_POINT('Origin',(0.,0.,-60.));
#53665=CARTESIAN_POINT('Origin',(1.79430359459332E-10,2.24999999982085,
-59.9999999997029));
#53666=CARTESIAN_POINT('Origin',(0.,22.,0.));
#53667=CARTESIAN_POINT('',(-6.73555739531044E-16,13.,-5.5));
#53668=CARTESIAN_POINT('Origin',(0.,13.,0.));
#53669=CARTESIAN_POINT('',(-6.73555739531044E-16,22.,-5.5));
#53670=CARTESIAN_POINT('',(-6.73555739531044E-16,22.,-5.5));
#53671=CARTESIAN_POINT('Origin',(0.,22.,0.));
#53672=CARTESIAN_POINT('Origin',(0.,22.,0.));
#53673=CARTESIAN_POINT('',(-1.75,0.500000000000001,3.03108891324553));
#53674=CARTESIAN_POINT('',(1.75,0.5,3.03108891324544));
#53675=CARTESIAN_POINT('Origin',(0.,0.5,0.));
#53676=CARTESIAN_POINT('',(-2.25,0.,2.68095132369089));
#53677=CARTESIAN_POINT('Origin',(6.82837120180579E-11,2.25000000006793,
-9.89575088539141E-11));
#53678=CARTESIAN_POINT('',(-2.25,0.,-2.68095132369089));
#53679=CARTESIAN_POINT('Origin',(0.,0.,0.));
#53680=CARTESIAN_POINT('',(-1.75,0.500000000000001,-3.03108891324553));
#53681=CARTESIAN_POINT('Origin',(1.41059108837993E-10,2.25000000014086,
2.02939887117282E-10));
#53682=CARTESIAN_POINT('',(-4.28626379701573E-16,0.499999999999998,-3.5));
#53683=CARTESIAN_POINT('Origin',(0.,0.5,0.));
#53684=CARTESIAN_POINT('',(-4.28626379701573E-16,13.,-3.5));
#53685=CARTESIAN_POINT('',(-4.28626379701573E-16,22.,-3.5));
#53686=CARTESIAN_POINT('Origin',(0.,13.,0.));
#53687=CARTESIAN_POINT('',(1.75,0.5,-3.03108891324566));
#53688=CARTESIAN_POINT('Origin',(0.,0.5,0.));
#53689=CARTESIAN_POINT('',(2.24999999999999,0.,-2.6809513236909));
#53690=CARTESIAN_POINT('Origin',(-1.22898358156931E-10,2.25000000012316,
9.97296689675409E-11));
#53691=CARTESIAN_POINT('',(2.24999999999999,0.,2.6809513236909));
#53692=CARTESIAN_POINT('Origin',(0.,0.,0.));
#53693=CARTESIAN_POINT('Origin',(1.95984894979517E-11,2.24999999998063,
-2.54418708323101E-11));
#53694=CARTESIAN_POINT('Origin',(-2.25,-1.4389599889981E-16,-450.));
#53695=CARTESIAN_POINT('',(-1.75,0.5,-450.));
#53696=CARTESIAN_POINT('',(-1.75,0.5,-450.));
#53697=CARTESIAN_POINT('',(-2.25,-1.4389599889981E-16,-450.));
#53698=CARTESIAN_POINT('',(-2.25,-1.4389599889981E-16,-450.));
#53699=CARTESIAN_POINT('',(-2.25,-1.4389599889981E-16,-450.));
#53700=CARTESIAN_POINT('Origin',(-1.75,0.5,-450.));
#53701=CARTESIAN_POINT('',(-1.75,0.5,-450.));
#53702=CARTESIAN_POINT('',(1.75,0.5,-450.));
#53703=CARTESIAN_POINT('Origin',(1.75,0.5,-450.));
#53704=CARTESIAN_POINT('',(2.25,-1.30104260698261E-15,-450.));
#53705=CARTESIAN_POINT('Origin',(0.,0.,-450.));
#53706=CARTESIAN_POINT('',(-2.25,-1.4389599889981E-16,-450.));
#53707=CARTESIAN_POINT('',(-2.25,-1.4389599889981E-16,-450.));
#53708=CARTESIAN_POINT('',(-2.25,-1.4389599889981E-16,-450.));
#53709=CARTESIAN_POINT('',(-2.25,-1.4389599889981E-16,-450.));
#53710=CARTESIAN_POINT('',(-2.25,-1.4389599889981E-16,-450.));
#53711=CARTESIAN_POINT('',(-2.25,-1.4389599889981E-16,-450.));
#53712=CARTESIAN_POINT('',(-2.25,-1.4389599889981E-16,-450.));
#53713=CARTESIAN_POINT('',(-2.25,-1.4389599889981E-16,30.));
#53714=CARTESIAN_POINT('',(-2.25,-1.4389599889981E-16,-450.));
#53715=CARTESIAN_POINT('',(-10.5,-1.28587913910472E-15,30.));
#53716=CARTESIAN_POINT('',(0.,0.,30.));
#53717=CARTESIAN_POINT('',(-10.5,-1.28587913910472E-15,-450.));
#53718=CARTESIAN_POINT('',(-10.5,-1.28587913910472E-15,-450.));
#53719=CARTESIAN_POINT('',(0.,0.,-450.));
#53720=CARTESIAN_POINT('Origin',(0.,0.,-450.));
#53721=CARTESIAN_POINT('',(2.24999999999999,2.75545529808154E-16,-450.));
#53722=CARTESIAN_POINT('',(2.25,-1.30104260698261E-15,-450.));
#53723=CARTESIAN_POINT('',(10.5,-1.28587913910472E-15,-450.));
#53724=CARTESIAN_POINT('',(0.,0.,-450.));
#53725=CARTESIAN_POINT('',(10.5,-1.28587913910472E-15,30.));
#53726=CARTESIAN_POINT('',(10.5,-1.28587913910472E-15,-450.));
#53727=CARTESIAN_POINT('',(2.25,-1.30104260698261E-15,30.));
#53728=CARTESIAN_POINT('',(0.,0.,30.));
#53729=CARTESIAN_POINT('',(2.25,-1.30104260698261E-15,-450.));
#53730=CARTESIAN_POINT('',(2.25,-1.30104260698261E-15,-450.));
#53731=CARTESIAN_POINT('',(2.25,-1.30104260698261E-15,-450.));
#53732=CARTESIAN_POINT('',(2.25,-1.30104260698261E-15,-450.));
#53733=CARTESIAN_POINT('',(2.25,-1.30104260698261E-15,-450.));
#53734=CARTESIAN_POINT('',(2.25,-1.30104260698261E-15,-450.));
#53735=CARTESIAN_POINT('',(2.25,-1.30104260698261E-15,-450.));
#53736=CARTESIAN_POINT('Origin',(-2.25,-1.4389599889981E-16,-450.));
#53737=CARTESIAN_POINT('Origin',(-1.75,0.5,-450.));
#53738=CARTESIAN_POINT('',(-1.75,0.5,-450.));
#53739=CARTESIAN_POINT('',(1.75,0.5,-450.));
#53740=CARTESIAN_POINT('Origin',(1.75,0.5,-450.));
#53741=CARTESIAN_POINT('Origin',(-2.25,-1.4389599889981E-16,-450.));
#53742=CARTESIAN_POINT('Origin',(-1.75,0.5,-450.));
#53743=CARTESIAN_POINT('',(-1.75,0.5,-450.));
#53744=CARTESIAN_POINT('',(1.75,0.5,-450.));
#53745=CARTESIAN_POINT('Origin',(1.75,0.5,-450.));
#53746=CARTESIAN_POINT('Origin',(-2.25,-1.4389599889981E-16,-450.));
#53747=CARTESIAN_POINT('Origin',(1.75,0.5,-450.));
#53748=CARTESIAN_POINT('',(1.75,0.5,-450.));
#53749=CARTESIAN_POINT('Origin',(-1.75,0.5,-450.));
#53750=CARTESIAN_POINT('',(-1.75,0.5,-450.));
#53751=CARTESIAN_POINT('Origin',(-2.25,-1.4389599889981E-16,-450.));
#53752=CARTESIAN_POINT('Origin',(-1.75,0.5,-450.));
#53753=CARTESIAN_POINT('',(-1.75,0.5,-450.));
#53754=CARTESIAN_POINT('',(1.75,0.5,-450.));
#53755=CARTESIAN_POINT('Origin',(1.75,0.5,-450.));
#53756=CARTESIAN_POINT('Origin',(-2.25,-1.4389599889981E-16,-450.));
#53757=CARTESIAN_POINT('Origin',(-1.75,0.5,-450.));
#53758=CARTESIAN_POINT('',(-1.75,0.5,-450.));
#53759=CARTESIAN_POINT('',(1.75,0.5,-450.));
#53760=CARTESIAN_POINT('Origin',(1.75,0.5,-450.));
#53761=CARTESIAN_POINT('Origin',(-2.25,-1.4389599889981E-16,-450.));
#53762=CARTESIAN_POINT('Origin',(-1.75,0.5,-450.));
#53763=CARTESIAN_POINT('',(-1.75,0.5,-450.));
#53764=CARTESIAN_POINT('',(1.75,0.5,-450.));
#53765=CARTESIAN_POINT('Origin',(1.75,0.5,-450.));
#53766=CARTESIAN_POINT('Origin',(-2.25,-1.4389599889981E-16,-450.));
#53767=CARTESIAN_POINT('Origin',(-1.75,0.5,-450.));
#53768=CARTESIAN_POINT('',(-1.75,0.5,30.));
#53769=CARTESIAN_POINT('',(-1.75,0.5,-450.));
#53770=CARTESIAN_POINT('',(1.75,0.5,30.));
#53771=CARTESIAN_POINT('',(1.75,0.5,-450.));
#53772=CARTESIAN_POINT('',(-1.75,0.5,30.));
#53773=CARTESIAN_POINT('Origin',(1.75,0.5,-450.));
#53774=CARTESIAN_POINT('',(1.75,0.5,30.));
#53775=CARTESIAN_POINT('Origin',(0.,0.,-450.));
#53776=CARTESIAN_POINT('',(-11.5,1.00000000000001,-450.));
#53777=CARTESIAN_POINT('',(-10.5,-1.28587913910472E-15,-450.));
#53778=CARTESIAN_POINT('',(-11.5,5.8257864376269,-450.));
#53779=CARTESIAN_POINT('',(-11.5,1.00000000000001,-450.));
#53780=CARTESIAN_POINT('',(-11.2071067811865,6.53289321881345,-450.));
#53781=CARTESIAN_POINT('Origin',(-10.5,5.8257864376269,-450.));
#53782=CARTESIAN_POINT('',(-8.19644660940673,9.54355339059324,-450.));
#53783=CARTESIAN_POINT('',(-11.5,6.24,-450.));
#53784=CARTESIAN_POINT('',(-8.05,9.89710678118651,-450.));
#53785=CARTESIAN_POINT('Origin',(-8.55,9.89710678118651,-450.));
#53786=CARTESIAN_POINT('',(-8.05,13.5928932188135,-450.));
#53787=CARTESIAN_POINT('',(-8.05,9.68999999999997,-450.));
#53788=CARTESIAN_POINT('',(-8.19644660940672,13.9464466094067,-450.));
#53789=CARTESIAN_POINT('Origin',(-8.55,13.5928932188135,-450.));
#53790=CARTESIAN_POINT('',(-8.57259699813414,14.3225969981341,-450.));
#53791=CARTESIAN_POINT('',(-8.05,13.8,-450.));
#53792=CARTESIAN_POINT('',(-8.71475010619428,14.6107663907404,-450.));
#53793=CARTESIAN_POINT('Origin',(-8.21904360754086,14.6761503887274,-450.));
#53794=CARTESIAN_POINT('',(-10.6942336092596,16.5902498938057,-450.));
#53795=CARTESIAN_POINT('Origin',(-10.995,14.31,-450.));
#53796=CARTESIAN_POINT('',(-10.9824030018658,16.7324030018659,-450.));
#53797=CARTESIAN_POINT('Origin',(-10.6288496112726,17.0859563924591,-450.));
#53798=CARTESIAN_POINT('',(-11.3535533905933,17.1035533905933,-450.));
#53799=CARTESIAN_POINT('',(-8.05,13.8,-450.));
#53800=CARTESIAN_POINT('',(-11.5,17.4571067811866,-450.));
#53801=CARTESIAN_POINT('Origin',(-11.,17.4571067811866,-450.));
#53802=CARTESIAN_POINT('',(-11.5,18.3428932188135,-450.));
#53803=CARTESIAN_POINT('',(-11.5,18.55,-450.));
#53804=CARTESIAN_POINT('',(-11.3535533905933,18.6964466094068,-450.));
#53805=CARTESIAN_POINT('Origin',(-11.,18.3428932188135,-450.));
#53806=CARTESIAN_POINT('',(-10.9824030018659,19.0675969981341,-450.));
#53807=CARTESIAN_POINT('',(-8.05,22.,-450.));
#53808=CARTESIAN_POINT('',(-10.6942336092596,19.2097501061943,-450.));
#53809=CARTESIAN_POINT('Origin',(-10.6288496112726,18.7140436075409,-450.));
#53810=CARTESIAN_POINT('',(-8.71475010619428,21.1892336092596,-450.));
#53811=CARTESIAN_POINT('Origin',(-10.995,21.49,-450.));
#53812=CARTESIAN_POINT('',(-8.57259699813413,21.4774030018659,-450.));
#53813=CARTESIAN_POINT('Origin',(-8.21904360754086,21.1238496112726,-450.));
#53814=CARTESIAN_POINT('',(-8.05,22.,-450.));
#53815=CARTESIAN_POINT('',(-8.05,22.,-450.));
#53816=CARTESIAN_POINT('',(8.05,22.,-450.));
#53817=CARTESIAN_POINT('',(-8.05,22.,-450.));
#53818=CARTESIAN_POINT('',(8.57259699813413,21.4774030018659,-450.));
#53819=CARTESIAN_POINT('',(8.05,22.,-450.));
#53820=CARTESIAN_POINT('',(8.71475010619428,21.1892336092596,-450.));
#53821=CARTESIAN_POINT('Origin',(8.21904360754086,21.1238496112726,-450.));
#53822=CARTESIAN_POINT('',(10.6942336092596,19.2097501061943,-450.));
#53823=CARTESIAN_POINT('Origin',(10.995,21.49,-450.));
#53824=CARTESIAN_POINT('',(10.9824030018659,19.0675969981341,-450.));
#53825=CARTESIAN_POINT('Origin',(10.6288496112726,18.7140436075409,-450.));
#53826=CARTESIAN_POINT('',(11.3535533905933,18.6964466094068,-450.));
#53827=CARTESIAN_POINT('',(8.05,22.,-450.));
#53828=CARTESIAN_POINT('',(11.5,18.3428932188135,-450.));
#53829=CARTESIAN_POINT('Origin',(11.,18.3428932188135,-450.));
#53830=CARTESIAN_POINT('',(11.5,17.4571067811866,-450.));
#53831=CARTESIAN_POINT('',(11.5,18.55,-450.));
#53832=CARTESIAN_POINT('',(11.3535533905933,17.1035533905933,-450.));
#53833=CARTESIAN_POINT('Origin',(11.,17.4571067811866,-450.));
#53834=CARTESIAN_POINT('',(10.9824030018658,16.7324030018659,-450.));
#53835=CARTESIAN_POINT('',(8.05,13.8,-450.));
#53836=CARTESIAN_POINT('',(10.6942336092596,16.5902498938057,-450.));
#53837=CARTESIAN_POINT('Origin',(10.6288496112726,17.0859563924591,-450.));
#53838=CARTESIAN_POINT('',(8.71475010619428,14.6107663907404,-450.));
#53839=CARTESIAN_POINT('Origin',(10.995,14.31,-450.));
#53840=CARTESIAN_POINT('',(8.57259699813414,14.3225969981341,-450.));
#53841=CARTESIAN_POINT('Origin',(8.21904360754086,14.6761503887274,-450.));
#53842=CARTESIAN_POINT('',(8.19644660940672,13.9464466094067,-450.));
#53843=CARTESIAN_POINT('',(8.05,13.8,-450.));
#53844=CARTESIAN_POINT('',(8.05,13.5928932188135,-450.));
#53845=CARTESIAN_POINT('Origin',(8.55,13.5928932188135,-450.));
#53846=CARTESIAN_POINT('',(8.05,9.89710678118651,-450.));
#53847=CARTESIAN_POINT('',(8.05,9.68999999999997,-450.));
#53848=CARTESIAN_POINT('',(8.19644660940673,9.54355339059324,-450.));
#53849=CARTESIAN_POINT('Origin',(8.55,9.89710678118651,-450.));
#53850=CARTESIAN_POINT('',(11.2071067811865,6.53289321881345,-450.));
#53851=CARTESIAN_POINT('',(11.5,6.24,-450.));
#53852=CARTESIAN_POINT('',(11.5,5.8257864376269,-450.));
#53853=CARTESIAN_POINT('Origin',(10.5,5.8257864376269,-450.));
#53854=CARTESIAN_POINT('',(11.5,1.00000000000001,-450.));
#53855=CARTESIAN_POINT('',(11.5,1.00000000000001,-450.));
#53856=CARTESIAN_POINT('',(10.5,-1.28587913910472E-15,-450.));
#53857=CARTESIAN_POINT('',(1.75,0.5,-450.));
#53858=CARTESIAN_POINT('',(1.75,0.5,-450.));
#53859=CARTESIAN_POINT('',(-1.75,0.5,-450.));
#53860=CARTESIAN_POINT('Origin',(0.,0.,30.));
#53861=CARTESIAN_POINT('',(-2.25,-1.4389599889981E-16,30.));
#53862=CARTESIAN_POINT('',(11.5,1.00000000000001,30.));
#53863=CARTESIAN_POINT('',(10.5,-1.28587913910472E-15,30.));
#53864=CARTESIAN_POINT('',(11.5,5.8257864376269,30.));
#53865=CARTESIAN_POINT('',(11.5,1.00000000000001,30.));
#53866=CARTESIAN_POINT('',(11.2071067811865,6.53289321881345,30.));
#53867=CARTESIAN_POINT('Origin',(10.5,5.8257864376269,30.));
#53868=CARTESIAN_POINT('',(8.19644660940673,9.54355339059324,30.));
#53869=CARTESIAN_POINT('',(11.5,6.24,30.));
#53870=CARTESIAN_POINT('',(8.05,9.89710678118651,30.));
#53871=CARTESIAN_POINT('Origin',(8.55,9.89710678118651,30.));
#53872=CARTESIAN_POINT('',(8.05,13.5928932188135,30.));
#53873=CARTESIAN_POINT('',(8.05,9.68999999999997,30.));
#53874=CARTESIAN_POINT('',(8.19644660940672,13.9464466094067,30.));
#53875=CARTESIAN_POINT('Origin',(8.55,13.5928932188135,30.));
#53876=CARTESIAN_POINT('',(8.57259699813414,14.3225969981341,30.));
#53877=CARTESIAN_POINT('',(8.05,13.8,30.));
#53878=CARTESIAN_POINT('',(8.71475010619428,14.6107663907404,30.));
#53879=CARTESIAN_POINT('Origin',(8.21904360754086,14.6761503887274,30.));
#53880=CARTESIAN_POINT('',(10.6942336092596,16.5902498938057,30.));
#53881=CARTESIAN_POINT('Origin',(10.995,14.31,30.));
#53882=CARTESIAN_POINT('',(10.9824030018658,16.7324030018659,30.));
#53883=CARTESIAN_POINT('Origin',(10.6288496112726,17.0859563924591,30.));
#53884=CARTESIAN_POINT('',(11.3535533905933,17.1035533905933,30.));
#53885=CARTESIAN_POINT('',(8.05,13.8,30.));
#53886=CARTESIAN_POINT('',(11.5,17.4571067811866,30.));
#53887=CARTESIAN_POINT('Origin',(11.,17.4571067811866,30.));
#53888=CARTESIAN_POINT('',(11.5,18.3428932188135,30.));
#53889=CARTESIAN_POINT('',(11.5,18.55,30.));
#53890=CARTESIAN_POINT('',(11.3535533905933,18.6964466094068,30.));
#53891=CARTESIAN_POINT('Origin',(11.,18.3428932188135,30.));
#53892=CARTESIAN_POINT('',(10.9824030018659,19.0675969981341,30.));
#53893=CARTESIAN_POINT('',(8.05,22.,30.));
#53894=CARTESIAN_POINT('',(10.6942336092596,19.2097501061943,30.));
#53895=CARTESIAN_POINT('Origin',(10.6288496112726,18.7140436075409,30.));
#53896=CARTESIAN_POINT('',(8.71475010619428,21.1892336092596,30.));
#53897=CARTESIAN_POINT('Origin',(10.995,21.49,30.));
#53898=CARTESIAN_POINT('',(8.57259699813413,21.4774030018659,30.));
#53899=CARTESIAN_POINT('Origin',(8.21904360754086,21.1238496112726,30.));
#53900=CARTESIAN_POINT('',(8.05,22.,30.));
#53901=CARTESIAN_POINT('',(8.05,22.,30.));
#53902=CARTESIAN_POINT('',(-8.05,22.,30.));
#53903=CARTESIAN_POINT('',(-8.05,22.,30.));
#53904=CARTESIAN_POINT('',(-8.57259699813413,21.4774030018659,30.));
#53905=CARTESIAN_POINT('',(-8.05,22.,30.));
#53906=CARTESIAN_POINT('',(-8.71475010619428,21.1892336092596,30.));
#53907=CARTESIAN_POINT('Origin',(-8.21904360754086,21.1238496112726,30.));
#53908=CARTESIAN_POINT('',(-10.6942336092596,19.2097501061943,30.));
#53909=CARTESIAN_POINT('Origin',(-10.995,21.49,30.));
#53910=CARTESIAN_POINT('',(-10.9824030018659,19.0675969981341,30.));
#53911=CARTESIAN_POINT('Origin',(-10.6288496112726,18.7140436075409,30.));
#53912=CARTESIAN_POINT('',(-11.3535533905933,18.6964466094068,30.));
#53913=CARTESIAN_POINT('',(-8.05,22.,30.));
#53914=CARTESIAN_POINT('',(-11.5,18.3428932188135,30.));
#53915=CARTESIAN_POINT('Origin',(-11.,18.3428932188135,30.));
#53916=CARTESIAN_POINT('',(-11.5,17.4571067811866,30.));
#53917=CARTESIAN_POINT('',(-11.5,18.55,30.));
#53918=CARTESIAN_POINT('',(-11.3535533905933,17.1035533905933,30.));
#53919=CARTESIAN_POINT('Origin',(-11.,17.4571067811866,30.));
#53920=CARTESIAN_POINT('',(-10.9824030018658,16.7324030018659,30.));
#53921=CARTESIAN_POINT('',(-8.05,13.8,30.));
#53922=CARTESIAN_POINT('',(-10.6942336092596,16.5902498938057,30.));
#53923=CARTESIAN_POINT('Origin',(-10.6288496112726,17.0859563924591,30.));
#53924=CARTESIAN_POINT('',(-8.71475010619428,14.6107663907404,30.));
#53925=CARTESIAN_POINT('Origin',(-10.995,14.31,30.));
#53926=CARTESIAN_POINT('',(-8.57259699813414,14.3225969981341,30.));
#53927=CARTESIAN_POINT('Origin',(-8.21904360754086,14.6761503887274,30.));
#53928=CARTESIAN_POINT('',(-8.19644660940672,13.9464466094067,30.));
#53929=CARTESIAN_POINT('',(-8.05,13.8,30.));
#53930=CARTESIAN_POINT('',(-8.05,13.5928932188135,30.));
#53931=CARTESIAN_POINT('Origin',(-8.55,13.5928932188135,30.));
#53932=CARTESIAN_POINT('',(-8.05,9.89710678118651,30.));
#53933=CARTESIAN_POINT('',(-8.05,9.68999999999997,30.));
#53934=CARTESIAN_POINT('',(-8.19644660940673,9.54355339059324,30.));
#53935=CARTESIAN_POINT('Origin',(-8.55,9.89710678118651,30.));
#53936=CARTESIAN_POINT('',(-11.2071067811865,6.53289321881345,30.));
#53937=CARTESIAN_POINT('',(-11.5,6.24,30.));
#53938=CARTESIAN_POINT('',(-11.5,5.8257864376269,30.));
#53939=CARTESIAN_POINT('Origin',(-10.5,5.8257864376269,30.));
#53940=CARTESIAN_POINT('',(-11.5,1.00000000000001,30.));
#53941=CARTESIAN_POINT('',(-11.5,1.00000000000001,30.));
#53942=CARTESIAN_POINT('',(-10.5,-1.28587913910472E-15,30.));
#53943=CARTESIAN_POINT('Origin',(8.05,13.8,-450.));
#53944=CARTESIAN_POINT('',(8.19644660940672,13.9464466094067,-450.));
#53945=CARTESIAN_POINT('',(8.57259699813414,14.3225969981341,30.));
#53946=CARTESIAN_POINT('Origin',(8.05,13.8,-450.));
#53947=CARTESIAN_POINT('',(11.3535533905933,17.1035533905933,-450.));
#53948=CARTESIAN_POINT('',(10.9824030018658,16.7324030018659,-450.));
#53949=CARTESIAN_POINT('Origin',(8.05,22.,-450.));
#53950=CARTESIAN_POINT('',(10.9824030018659,19.0675969981341,30.));
#53951=CARTESIAN_POINT('',(11.3535533905933,18.6964466094068,-450.));
#53952=CARTESIAN_POINT('Origin',(8.05,22.,-450.));
#53953=CARTESIAN_POINT('',(8.57259699813413,21.4774030018659,-450.));
#53954=CARTESIAN_POINT('',(8.05,22.,-450.));
#53955=CARTESIAN_POINT('Origin',(-8.05,13.8,-450.));
#53956=CARTESIAN_POINT('',(-8.19644660940672,13.9464466094067,30.));
#53957=CARTESIAN_POINT('',(-8.57259699813414,14.3225969981341,-450.));
#53958=CARTESIAN_POINT('Origin',(-8.05,22.,-450.));
#53959=CARTESIAN_POINT('',(-10.9824030018659,19.0675969981341,-450.));
#53960=CARTESIAN_POINT('',(-11.3535533905933,18.6964466094068,-450.));
#53961=CARTESIAN_POINT('Origin',(-8.05,22.,-450.));
#53962=CARTESIAN_POINT('',(-8.05,22.,-450.));
#53963=CARTESIAN_POINT('Origin',(-10.5,-1.28587913910472E-15,-450.));
#53964=CARTESIAN_POINT('',(-11.5,1.00000000000001,-450.));
#53965=CARTESIAN_POINT('Origin',(-11.5,1.00000000000001,-450.));
#53966=CARTESIAN_POINT('',(-11.5,5.8257864376269,-450.));
#53967=CARTESIAN_POINT('Origin',(-11.5,6.24,-450.));
#53968=CARTESIAN_POINT('',(-11.2071067811865,6.53289321881345,-450.));
#53969=CARTESIAN_POINT('',(-8.19644660940673,9.54355339059324,-450.));
#53970=CARTESIAN_POINT('Origin',(-8.05,9.68999999999997,-450.));
#53971=CARTESIAN_POINT('',(-8.05,9.89710678118651,30.));
#53972=CARTESIAN_POINT('',(-8.05,13.5928932188135,-450.));
#53973=CARTESIAN_POINT('Origin',(-8.05,13.8,-450.));
#53974=CARTESIAN_POINT('',(-11.3535533905933,17.1035533905933,-450.));
#53975=CARTESIAN_POINT('',(-10.9824030018658,16.7324030018659,30.));
#53976=CARTESIAN_POINT('Origin',(-11.5,18.55,-450.));
#53977=CARTESIAN_POINT('',(-11.5,18.3428932188135,-450.));
#53978=CARTESIAN_POINT('',(-11.5,17.4571067811866,-450.));
#53979=CARTESIAN_POINT('Origin',(-8.05,22.,-450.));
#53980=CARTESIAN_POINT('',(-8.57259699813413,21.4774030018659,30.));
#53981=CARTESIAN_POINT('Origin',(-10.995,21.49,-450.));
#53982=CARTESIAN_POINT('',(-10.6942336092596,19.2097501061943,-450.));
#53983=CARTESIAN_POINT('',(-8.71475010619428,21.1892336092596,-450.));
#53984=CARTESIAN_POINT('Origin',(-10.995,14.31,-450.));
#53985=CARTESIAN_POINT('',(-10.6942336092596,16.5902498938057,-450.));
#53986=CARTESIAN_POINT('',(-8.71475010619428,14.6107663907404,-450.));
#53987=CARTESIAN_POINT('Origin',(-10.6288496112726,18.7140436075409,-450.));
#53988=CARTESIAN_POINT('Origin',(-11.,18.3428932188135,-450.));
#53989=CARTESIAN_POINT('Origin',(-11.,17.4571067811866,-450.));
#53990=CARTESIAN_POINT('Origin',(-10.6288496112726,17.0859563924591,-450.));
#53991=CARTESIAN_POINT('Origin',(-8.55,9.89710678118651,-450.));
#53992=CARTESIAN_POINT('Origin',(-8.55,13.5928932188135,-450.));
#53993=CARTESIAN_POINT('Origin',(-8.21904360754086,14.6761503887274,-450.));
#53994=CARTESIAN_POINT('Origin',(-8.21904360754086,21.1238496112726,-450.));
#53995=CARTESIAN_POINT('Origin',(-10.5,5.8257864376269,-450.));
#53996=CARTESIAN_POINT('Origin',(11.5,18.55,-450.));
#53997=CARTESIAN_POINT('',(11.5,18.3428932188135,-450.));
#53998=CARTESIAN_POINT('',(11.5,17.4571067811866,-450.));
#53999=CARTESIAN_POINT('Origin',(8.05,9.68999999999997,-450.));
#54000=CARTESIAN_POINT('',(8.05,9.89710678118651,-450.));
#54001=CARTESIAN_POINT('',(8.05,13.5928932188135,30.));
#54002=CARTESIAN_POINT('Origin',(11.5,6.24,-450.));
#54003=CARTESIAN_POINT('',(11.2071067811865,6.53289321881345,-450.));
#54004=CARTESIAN_POINT('',(8.19644660940673,9.54355339059324,30.));
#54005=CARTESIAN_POINT('Origin',(11.5,1.00000000000001,-450.));
#54006=CARTESIAN_POINT('',(11.5,5.8257864376269,-450.));
#54007=CARTESIAN_POINT('',(11.5,1.00000000000001,-450.));
#54008=CARTESIAN_POINT('Origin',(10.5,-1.28587913910472E-15,-450.));
#54009=CARTESIAN_POINT('Origin',(10.995,21.49,-450.));
#54010=CARTESIAN_POINT('',(10.6942336092596,19.2097501061943,-450.));
#54011=CARTESIAN_POINT('',(8.71475010619428,21.1892336092596,-450.));
#54012=CARTESIAN_POINT('Origin',(10.995,14.31,-450.));
#54013=CARTESIAN_POINT('',(10.6942336092596,16.5902498938057,-450.));
#54014=CARTESIAN_POINT('',(8.71475010619428,14.6107663907404,-450.));
#54015=CARTESIAN_POINT('Origin',(10.6288496112726,18.7140436075409,-450.));
#54016=CARTESIAN_POINT('Origin',(11.,18.3428932188135,-450.));
#54017=CARTESIAN_POINT('Origin',(11.,17.4571067811866,-450.));
#54018=CARTESIAN_POINT('Origin',(10.6288496112726,17.0859563924591,-450.));
#54019=CARTESIAN_POINT('Origin',(8.55,9.89710678118651,-450.));
#54020=CARTESIAN_POINT('Origin',(8.55,13.5928932188135,-450.));
#54021=CARTESIAN_POINT('Origin',(8.21904360754086,14.6761503887274,-450.));
#54022=CARTESIAN_POINT('Origin',(8.21904360754086,21.1238496112726,-450.));
#54023=CARTESIAN_POINT('Origin',(10.5,5.8257864376269,-450.));
#54024=CARTESIAN_POINT('Origin',(-2.25,-1.4389599889981E-16,-450.));
#54025=CARTESIAN_POINT('Origin',(-1.75,0.5,-450.));
#54026=CARTESIAN_POINT('',(1.75,0.5,-450.));
#54027=CARTESIAN_POINT('Origin',(1.75,0.5,-450.));
#54028=CARTESIAN_POINT('Origin',(3.5,13.,0.));
#54029=CARTESIAN_POINT('Origin',(3.5,13.,-60.));
#54030=CARTESIAN_POINT('Origin',(3.5,13.,-120.));
#54031=CARTESIAN_POINT('Origin',(3.5,13.,-180.));
#54032=CARTESIAN_POINT('Origin',(3.5,13.,-240.));
#54033=CARTESIAN_POINT('Origin',(3.5,13.,-300.));
#54034=CARTESIAN_POINT('Origin',(3.5,13.,-360.));
#54035=CARTESIAN_POINT('Origin',(3.5,13.,-420.));
#57031=UNCERTAINTY_MEASURE_WITH_UNIT(LENGTH_MEASURE(0.01),#57080,
'DISTANCE_ACCURACY_VALUE',
'Maximum model space distance between geometric entities at asserted c
onnectivities');
#57040=UNCERTAINTY_MEASURE_WITH_UNIT(LENGTH_MEASURE(0.01),#57080,
'DISTANCE_ACCURACY_VALUE',
'Maximum model space distance between geometric entities at asserted c
onnectivities');
#57070=(
GEOMETRIC_REPRESENTATION_CONTEXT(3)
GLOBAL_UNCERTAINTY_ASSIGNED_CONTEXT((#57031))
GLOBAL_UNIT_ASSIGNED_CONTEXT((#57080,#57082,#57083))
REPRESENTATION_CONTEXT('','3D')
);
#57079=(
GEOMETRIC_REPRESENTATION_CONTEXT(3)
GLOBAL_UNCERTAINTY_ASSIGNED_CONTEXT((#57040))
GLOBAL_UNIT_ASSIGNED_CONTEXT((#57080,#57082,#57083))
REPRESENTATION_CONTEXT('','3D')
);
#57080=(
LENGTH_UNIT()
NAMED_UNIT(*)
SI_UNIT(.MILLI.,.METRE.)
);
#57082=(
NAMED_UNIT(*)
PLANE_ANGLE_UNIT()
SI_UNIT($,.RADIAN.)
);
#57083=(
NAMED_UNIT(*)
SI_UNIT($,.STERADIAN.)
SOLID_ANGLE_UNIT()
);
#57113=SHAPE_DEFINITION_REPRESENTATION(#57167,#57278);
#57167=PRODUCT_DEFINITION_SHAPE('',$,#57317);
#57278=SHAPE_REPRESENTATION('',(#26270),#57070);
#57287=PRODUCT_DEFINITION_CONTEXT('part definition',#57403,'design');
#57317=PRODUCT_DEFINITION('Linear Guide Rail','Linear Guide Rail',#57355,
#57287);
#57355=PRODUCT_DEFINITION_FORMATION('',$,#57434);
#57403=APPLICATION_CONTEXT(
'Core Data for Automotive Mechanical Design Process');
#57404=PRODUCT_CONTEXT('part definition',#57403,'mechanical');
#57434=PRODUCT('Linear Guide Rail','Linear Guide Rail',$,(#57404));
#57444=PRESENTATION_STYLE_ASSIGNMENT((#57446));
#57446=SURFACE_STYLE_USAGE(.BOTH.,#57448);
#57448=SURFACE_SIDE_STYLE('',(#57450));
#57450=SURFACE_STYLE_FILL_AREA(#57452);
#57452=FILL_AREA_STYLE('Opaque(202,209,238)',(#57454));
#57454=FILL_AREA_STYLE_COLOUR('Opaque(202,209,238)',#57456);
#57456=COLOUR_RGB('Opaque(202,209,238)',0.792156862745098,0.819607843137255,
0.933333333333333);
ENDSEC;
END-ISO-10303-21;
